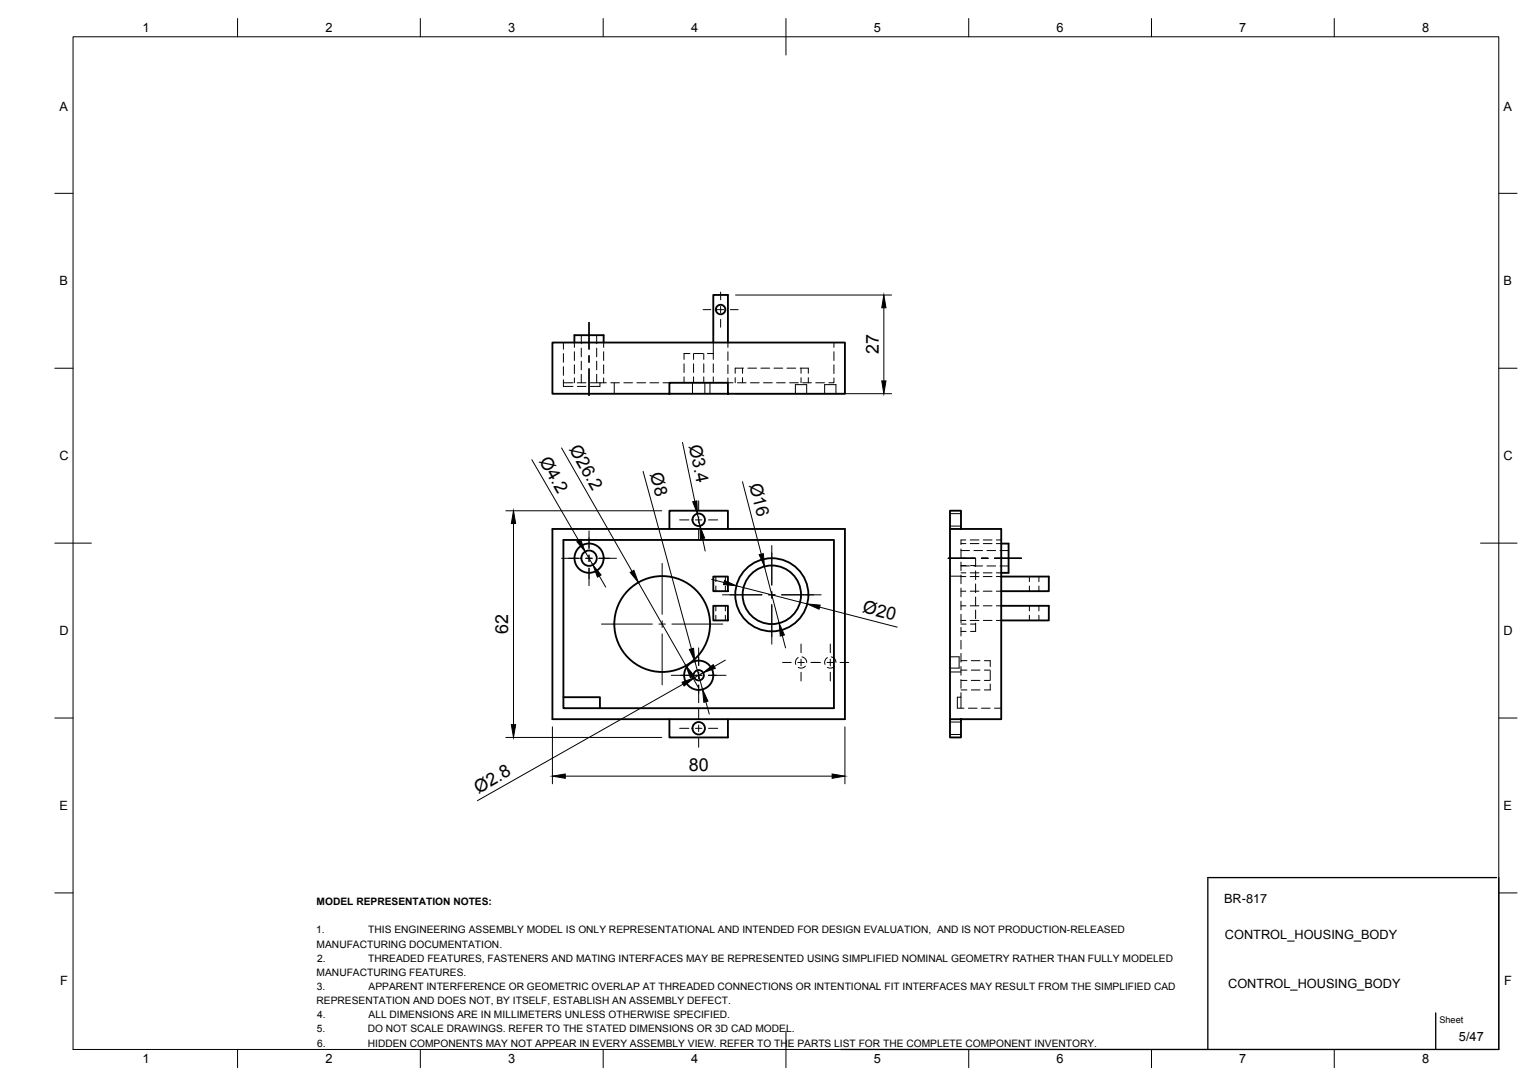
ISO-10303-21;
HEADER;
FILE_DESCRIPTION((''),'2;1');
FILE_NAME('CONTROL_HOUSING_BODY.step','2026-10-01T22:07:29-07:00',(''),(''),'','','');
FILE_SCHEMA (('AUTOMOTIVE_DESIGN { 1 0 10303 214 3 1 1 }'));
ENDSEC;
DATA;
#10=MECHANICAL_DESIGN_GEOMETRIC_PRESENTATION_REPRESENTATION('',(#543),#15484);
#473=SHAPE_REPRESENTATION_RELATIONSHIP('SRR','None',#15620,#508) ;
#508=ADVANCED_BREP_SHAPE_REPRESENTATION('',(#585),#15444) ;
#543=STYLED_ITEM('',(#15833),#585) ;
#585=MANIFOLD_SOLID_BREP('CONTROL_HOUSING_BODY',#8252) ;
#626=CYLINDRICAL_SURFACE('',#8695,0.155) ;
#627=CYLINDRICAL_SURFACE('',#8699,0.155) ;
#628=CYLINDRICAL_SURFACE('',#8703,0.17) ;
#629=CYLINDRICAL_SURFACE('',#8711,0.17) ;
#630=CYLINDRICAL_SURFACE('',#8719,0.14) ;
#631=CYLINDRICAL_SURFACE('',#8722,0.4) ;
#632=CYLINDRICAL_SURFACE('',#8726,0.8) ;
#633=CYLINDRICAL_SURFACE('',#8729,1.) ;
#634=CYLINDRICAL_SURFACE('',#8732,0.21) ;
#635=CYLINDRICAL_SURFACE('',#8735,0.4) ;
#636=CYLINDRICAL_SURFACE('',#8739,0.13) ;
#637=CYLINDRICAL_SURFACE('',#8742,0.13) ;
#638=CYLINDRICAL_SURFACE('',#8755,1.31) ;
#810=FACE_BOUND('',#1871,.T.) ;
#811=FACE_BOUND('',#1872,.T.) ;
#812=FACE_BOUND('',#1873,.T.) ;
#813=FACE_BOUND('',#1874,.T.) ;
#814=FACE_BOUND('',#1875,.T.) ;
#815=FACE_BOUND('',#1876,.T.) ;
#816=FACE_BOUND('',#1883,.T.) ;
#817=FACE_BOUND('',#1890,.T.) ;
#818=FACE_BOUND('',#1898,.T.) ;
#819=FACE_BOUND('',#1903,.T.) ;
#820=FACE_BOUND('',#1907,.T.) ;
#821=FACE_BOUND('',#1913,.T.) ;
#822=FACE_BOUND('',#1916,.T.) ;
#823=FACE_BOUND('',#1920,.T.) ;
#824=FACE_BOUND('',#1923,.T.) ;
#825=FACE_BOUND('',#1930,.T.) ;
#826=FACE_BOUND('',#1932,.T.) ;
#827=FACE_BOUND('',#1933,.T.) ;
#828=FACE_BOUND('',#1934,.T.) ;
#829=FACE_BOUND('',#1935,.T.) ;
#830=FACE_BOUND('',#1936,.T.) ;
#885=CIRCLE('',#8691,0.4) ;
#886=CIRCLE('',#8692,0.4) ;
#887=CIRCLE('',#8693,1.31) ;
#888=CIRCLE('',#8694,1.) ;
#889=CIRCLE('',#8696,0.155) ;
#890=CIRCLE('',#8697,0.155) ;
#891=CIRCLE('',#8700,0.155) ;
#892=CIRCLE('',#8701,0.155) ;
#893=CIRCLE('',#8704,0.17) ;
#894=CIRCLE('',#8705,0.17) ;
#895=CIRCLE('',#8712,0.17) ;
#896=CIRCLE('',#8713,0.17) ;
#897=CIRCLE('',#8720,0.14) ;
#898=CIRCLE('',#8721,0.14) ;
#899=CIRCLE('',#8723,0.4) ;
#900=CIRCLE('',#8727,0.8) ;
#901=CIRCLE('',#8728,0.8) ;
#902=CIRCLE('',#8730,1.) ;
#903=CIRCLE('',#8733,0.21) ;
#904=CIRCLE('',#8734,0.21) ;
#905=CIRCLE('',#8736,0.4) ;
#906=CIRCLE('',#8740,0.13) ;
#907=CIRCLE('',#8741,0.13) ;
#908=CIRCLE('',#8743,0.13) ;
#909=CIRCLE('',#8744,0.13) ;
#910=CIRCLE('',#8756,1.31) ;
#1365=FACE_OUTER_BOUND('',#1865,.T.) ;
#1366=FACE_OUTER_BOUND('',#1866,.T.) ;
#1367=FACE_OUTER_BOUND('',#1867,.T.) ;
#1368=FACE_OUTER_BOUND('',#1868,.T.) ;
#1369=FACE_OUTER_BOUND('',#1869,.T.) ;
#1370=FACE_OUTER_BOUND('',#1870,.T.) ;
#1371=FACE_OUTER_BOUND('',#1877,.T.) ;
#1372=FACE_OUTER_BOUND('',#1878,.T.) ;
#1373=FACE_OUTER_BOUND('',#1879,.T.) ;
#1374=FACE_OUTER_BOUND('',#1880,.T.) ;
#1375=FACE_OUTER_BOUND('',#1881,.T.) ;
#1376=FACE_OUTER_BOUND('',#1882,.T.) ;
#1377=FACE_OUTER_BOUND('',#1884,.T.) ;
#1378=FACE_OUTER_BOUND('',#1885,.T.) ;
#1379=FACE_OUTER_BOUND('',#1886,.T.) ;
#1380=FACE_OUTER_BOUND('',#1887,.T.) ;
#1381=FACE_OUTER_BOUND('',#1888,.T.) ;
#1382=FACE_OUTER_BOUND('',#1889,.T.) ;
#1383=FACE_OUTER_BOUND('',#1891,.T.) ;
#1384=FACE_OUTER_BOUND('',#1892,.T.) ;
#1385=FACE_OUTER_BOUND('',#1893,.T.) ;
#1386=FACE_OUTER_BOUND('',#1894,.T.) ;
#1387=FACE_OUTER_BOUND('',#1895,.T.) ;
#1388=FACE_OUTER_BOUND('',#1896,.T.) ;
#1389=FACE_OUTER_BOUND('',#1897,.T.) ;
#1390=FACE_OUTER_BOUND('',#1899,.T.) ;
#1391=FACE_OUTER_BOUND('',#1900,.T.) ;
#1392=FACE_OUTER_BOUND('',#1901,.T.) ;
#1393=FACE_OUTER_BOUND('',#1902,.T.) ;
#1394=FACE_OUTER_BOUND('',#1904,.T.) ;
#1395=FACE_OUTER_BOUND('',#1905,.T.) ;
#1396=FACE_OUTER_BOUND('',#1906,.T.) ;
#1397=FACE_OUTER_BOUND('',#1908,.T.) ;
#1398=FACE_OUTER_BOUND('',#1909,.T.) ;
#1399=FACE_OUTER_BOUND('',#1910,.T.) ;
#1400=FACE_OUTER_BOUND('',#1911,.T.) ;
#1401=FACE_OUTER_BOUND('',#1912,.T.) ;
#1402=FACE_OUTER_BOUND('',#1914,.T.) ;
#1403=FACE_OUTER_BOUND('',#1915,.T.) ;
#1404=FACE_OUTER_BOUND('',#1917,.T.) ;
#1405=FACE_OUTER_BOUND('',#1918,.T.) ;
#1406=FACE_OUTER_BOUND('',#1919,.T.) ;
#1407=FACE_OUTER_BOUND('',#1921,.T.) ;
#1408=FACE_OUTER_BOUND('',#1922,.T.) ;
#1409=FACE_OUTER_BOUND('',#1924,.T.) ;
#1410=FACE_OUTER_BOUND('',#1925,.T.) ;
#1411=FACE_OUTER_BOUND('',#1926,.T.) ;
#1412=FACE_OUTER_BOUND('',#1927,.T.) ;
#1413=FACE_OUTER_BOUND('',#1928,.T.) ;
#1414=FACE_OUTER_BOUND('',#1929,.T.) ;
#1415=FACE_OUTER_BOUND('',#1931,.T.) ;
#1416=FACE_OUTER_BOUND('',#1937,.T.) ;
#1417=FACE_OUTER_BOUND('',#1938,.T.) ;
#1865=EDGE_LOOP('',(#5273,#5274,#5275,#5276)) ;
#1866=EDGE_LOOP('',(#5277,#5278,#5279,#5280,#5281,#5282)) ;
#1867=EDGE_LOOP('',(#5283,#5284,#5285,#5286,#5287,#5288)) ;
#1868=EDGE_LOOP('',(#5289,#5290,#5291,#5292)) ;
#1869=EDGE_LOOP('',(#5293,#5294,#5295,#5296)) ;
#1870=EDGE_LOOP('',(#5297,#5298,#5299,#5300,#5301,#5302)) ;
#1871=EDGE_LOOP('',(#5303)) ;
#1872=EDGE_LOOP('',(#5304)) ;
#1873=EDGE_LOOP('',(#5305,#5306,#5307,#5308)) ;
#1874=EDGE_LOOP('',(#5309,#5310,#5311,#5312)) ;
#1875=EDGE_LOOP('',(#5313)) ;
#1876=EDGE_LOOP('',(#5314)) ;
#1877=EDGE_LOOP('',(#5315,#5316,#5317,#5318)) ;
#1878=EDGE_LOOP('',(#5319)) ;
#1879=EDGE_LOOP('',(#5320,#5321,#5322,#5323)) ;
#1880=EDGE_LOOP('',(#5324)) ;
#1881=EDGE_LOOP('',(#5325,#5326,#5327,#5328)) ;
#1882=EDGE_LOOP('',(#5329,#5330,#5331,#5332)) ;
#1883=EDGE_LOOP('',(#5333)) ;
#1884=EDGE_LOOP('',(#5334,#5335,#5336,#5337)) ;
#1885=EDGE_LOOP('',(#5338,#5339,#5340,#5341)) ;
#1886=EDGE_LOOP('',(#5342,#5343,#5344,#5345)) ;
#1887=EDGE_LOOP('',(#5346,#5347,#5348,#5349,#5350,#5351,#5352,#5353)) ;
#1888=EDGE_LOOP('',(#5354,#5355,#5356,#5357)) ;
#1889=EDGE_LOOP('',(#5358,#5359,#5360,#5361)) ;
#1890=EDGE_LOOP('',(#5362)) ;
#1891=EDGE_LOOP('',(#5363,#5364,#5365,#5366)) ;
#1892=EDGE_LOOP('',(#5367,#5368,#5369,#5370)) ;
#1893=EDGE_LOOP('',(#5371,#5372,#5373,#5374)) ;
#1894=EDGE_LOOP('',(#5375,#5376,#5377,#5378,#5379,#5380,#5381,#5382)) ;
#1895=EDGE_LOOP('',(#5383,#5384,#5385,#5386)) ;
#1896=EDGE_LOOP('',(#5387,#5388,#5389,#5390)) ;
#1897=EDGE_LOOP('',(#5391)) ;
#1898=EDGE_LOOP('',(#5392)) ;
#1899=EDGE_LOOP('',(#5393)) ;
#1900=EDGE_LOOP('',(#5394,#5395,#5396,#5397)) ;
#1901=EDGE_LOOP('',(#5398,#5399,#5400,#5401)) ;
#1902=EDGE_LOOP('',(#5402)) ;
#1903=EDGE_LOOP('',(#5403)) ;
#1904=EDGE_LOOP('',(#5404,#5405,#5406,#5407)) ;
#1905=EDGE_LOOP('',(#5408,#5409,#5410,#5411)) ;
#1906=EDGE_LOOP('',(#5412)) ;
#1907=EDGE_LOOP('',(#5413)) ;
#1908=EDGE_LOOP('',(#5414)) ;
#1909=EDGE_LOOP('',(#5415,#5416,#5417,#5418)) ;
#1910=EDGE_LOOP('',(#5419,#5420,#5421,#5422)) ;
#1911=EDGE_LOOP('',(#5423,#5424,#5425,#5426)) ;
#1912=EDGE_LOOP('',(#5427,#5428,#5429,#5430)) ;
#1913=EDGE_LOOP('',(#5431)) ;
#1914=EDGE_LOOP('',(#5432,#5433,#5434,#5435)) ;
#1915=EDGE_LOOP('',(#5436,#5437,#5438,#5439)) ;
#1916=EDGE_LOOP('',(#5440)) ;
#1917=EDGE_LOOP('',(#5441,#5442,#5443,#5444)) ;
#1918=EDGE_LOOP('',(#5445,#5446,#5447,#5448)) ;
#1919=EDGE_LOOP('',(#5449,#5450,#5451,#5452)) ;
#1920=EDGE_LOOP('',(#5453)) ;
#1921=EDGE_LOOP('',(#5454,#5455,#5456,#5457)) ;
#1922=EDGE_LOOP('',(#5458,#5459,#5460,#5461)) ;
#1923=EDGE_LOOP('',(#5462)) ;
#1924=EDGE_LOOP('',(#5463,#5464,#5465,#5466)) ;
#1925=EDGE_LOOP('',(#5467,#5468,#5469,#5470)) ;
#1926=EDGE_LOOP('',(#5471,#5472,#5473,#5474)) ;
#1927=EDGE_LOOP('',(#5475,#5476,#5477,#5478)) ;
#1928=EDGE_LOOP('',(#5479)) ;
#1929=EDGE_LOOP('',(#5480,#5481,#5482,#5483)) ;
#1930=EDGE_LOOP('',(#5484,#5485,#5486,#5487)) ;
#1931=EDGE_LOOP('',(#5488,#5489,#5490,#5491,#5492,#5493,#5494,#5495,#5496,
#5497,#5498,#5499)) ;
#1932=EDGE_LOOP('',(#5500)) ;
#1933=EDGE_LOOP('',(#5501)) ;
#1934=EDGE_LOOP('',(#5502)) ;
#1935=EDGE_LOOP('',(#5503)) ;
#1936=EDGE_LOOP('',(#5504)) ;
#1937=EDGE_LOOP('',(#5505,#5506,#5507,#5508)) ;
#1938=EDGE_LOOP('',(#5509,#5510,#5511,#5512)) ;
#2440=LINE('',#12891,#2914) ;
#2441=LINE('',#12893,#2915) ;
#2442=LINE('',#12895,#2916) ;
#2443=LINE('',#12896,#2917) ;
#2444=LINE('',#12899,#2918) ;
#2445=LINE('',#12901,#2919) ;
#2446=LINE('',#12903,#2920) ;
#2447=LINE('',#12905,#2921) ;
#2448=LINE('',#12906,#2922) ;
#2449=LINE('',#12909,#2923) ;
#2450=LINE('',#12911,#2924) ;
#2451=LINE('',#12913,#2925) ;
#2452=LINE('',#12914,#2926) ;
#2453=LINE('',#12917,#2927) ;
#2454=LINE('',#12918,#2928) ;
#2455=LINE('',#12920,#2929) ;
#2456=LINE('',#12923,#2930) ;
#2457=LINE('',#12924,#2931) ;
#2458=LINE('',#12931,#2932) ;
#2459=LINE('',#12933,#2933) ;
#2460=LINE('',#12935,#2934) ;
#2461=LINE('',#12936,#2935) ;
#2462=LINE('',#12939,#2936) ;
#2463=LINE('',#12941,#2937) ;
#2464=LINE('',#12943,#2938) ;
#2465=LINE('',#12944,#2939) ;
#2466=LINE('',#12953,#2940) ;
#2467=LINE('',#12960,#2941) ;
#2468=LINE('',#12967,#2942) ;
#2469=LINE('',#12972,#2943) ;
#2470=LINE('',#12974,#2944) ;
#2471=LINE('',#12976,#2945) ;
#2472=LINE('',#12977,#2946) ;
#2473=LINE('',#12980,#2947) ;
#2474=LINE('',#12982,#2948) ;
#2475=LINE('',#12983,#2949) ;
#2476=LINE('',#12986,#2950) ;
#2477=LINE('',#12987,#2951) ;
#2478=LINE('',#12990,#2952) ;
#2479=LINE('',#12991,#2953) ;
#2480=LINE('',#12994,#2954) ;
#2481=LINE('',#12996,#2955) ;
#2482=LINE('',#12998,#2956) ;
#2483=LINE('',#13000,#2957) ;
#2484=LINE('',#13001,#2958) ;
#2485=LINE('',#13006,#2959) ;
#2486=LINE('',#13011,#2960) ;
#2487=LINE('',#13013,#2961) ;
#2488=LINE('',#13015,#2962) ;
#2489=LINE('',#13016,#2963) ;
#2490=LINE('',#13019,#2964) ;
#2491=LINE('',#13021,#2965) ;
#2492=LINE('',#13022,#2966) ;
#2493=LINE('',#13025,#2967) ;
#2494=LINE('',#13026,#2968) ;
#2495=LINE('',#13029,#2969) ;
#2496=LINE('',#13030,#2970) ;
#2497=LINE('',#13033,#2971) ;
#2498=LINE('',#13035,#2972) ;
#2499=LINE('',#13037,#2973) ;
#2500=LINE('',#13039,#2974) ;
#2501=LINE('',#13040,#2975) ;
#2502=LINE('',#13045,#2976) ;
#2503=LINE('',#13050,#2977) ;
#2504=LINE('',#13057,#2978) ;
#2505=LINE('',#13062,#2979) ;
#2506=LINE('',#13068,#2980) ;
#2507=LINE('',#13073,#2981) ;
#2508=LINE('',#13080,#2982) ;
#2509=LINE('',#13086,#2983) ;
#2510=LINE('',#13091,#2984) ;
#2511=LINE('',#13093,#2985) ;
#2512=LINE('',#13095,#2986) ;
#2513=LINE('',#13096,#2987) ;
#2514=LINE('',#13098,#2988) ;
#2515=LINE('',#13099,#2989) ;
#2516=LINE('',#13101,#2990) ;
#2517=LINE('',#13103,#2991) ;
#2518=LINE('',#13108,#2992) ;
#2519=LINE('',#13110,#2993) ;
#2520=LINE('',#13112,#2994) ;
#2521=LINE('',#13113,#2995) ;
#2522=LINE('',#13115,#2996) ;
#2523=LINE('',#13116,#2997) ;
#2524=LINE('',#13118,#2998) ;
#2525=LINE('',#13120,#2999) ;
#2526=LINE('',#13125,#3000) ;
#2527=LINE('',#13128,#3001) ;
#2528=LINE('',#13129,#3002) ;
#2529=LINE('',#13131,#3003) ;
#2530=LINE('',#13134,#3004) ;
#2531=LINE('',#13135,#3005) ;
#2532=LINE('',#13137,#3006) ;
#2533=LINE('',#13138,#3007) ;
#2914=VECTOR('',#9933,1.) ;
#2915=VECTOR('',#9934,1.) ;
#2916=VECTOR('',#9935,1.) ;
#2917=VECTOR('',#9936,1.) ;
#2918=VECTOR('',#9939,1.) ;
#2919=VECTOR('',#9940,1.) ;
#2920=VECTOR('',#9941,1.) ;
#2921=VECTOR('',#9942,1.) ;
#2922=VECTOR('',#9943,1.) ;
#2923=VECTOR('',#9946,1.) ;
#2924=VECTOR('',#9947,1.) ;
#2925=VECTOR('',#9948,1.) ;
#2926=VECTOR('',#9949,1.) ;
#2927=VECTOR('',#9952,1.) ;
#2928=VECTOR('',#9953,1.) ;
#2929=VECTOR('',#9956,1.) ;
#2930=VECTOR('',#9959,1.) ;
#2931=VECTOR('',#9960,1.) ;
#2932=VECTOR('',#9965,1.) ;
#2933=VECTOR('',#9966,1.) ;
#2934=VECTOR('',#9967,1.) ;
#2935=VECTOR('',#9968,1.) ;
#2936=VECTOR('',#9969,1.) ;
#2937=VECTOR('',#9970,1.) ;
#2938=VECTOR('',#9971,1.) ;
#2939=VECTOR('',#9972,1.) ;
#2940=VECTOR('',#9981,0.155) ;
#2941=VECTOR('',#9990,0.155) ;
#2942=VECTOR('',#9999,0.17) ;
#2943=VECTOR('',#10004,1.) ;
#2944=VECTOR('',#10005,1.) ;
#2945=VECTOR('',#10006,1.) ;
#2946=VECTOR('',#10007,1.) ;
#2947=VECTOR('',#10010,1.) ;
#2948=VECTOR('',#10011,1.) ;
#2949=VECTOR('',#10012,1.) ;
#2950=VECTOR('',#10015,1.) ;
#2951=VECTOR('',#10016,1.) ;
#2952=VECTOR('',#10019,1.) ;
#2953=VECTOR('',#10020,1.) ;
#2954=VECTOR('',#10023,1.) ;
#2955=VECTOR('',#10024,1.) ;
#2956=VECTOR('',#10025,1.) ;
#2957=VECTOR('',#10026,1.) ;
#2958=VECTOR('',#10027,1.) ;
#2959=VECTOR('',#10032,0.17) ;
#2960=VECTOR('',#10037,1.) ;
#2961=VECTOR('',#10038,1.) ;
#2962=VECTOR('',#10039,1.) ;
#2963=VECTOR('',#10040,1.) ;
#2964=VECTOR('',#10043,1.) ;
#2965=VECTOR('',#10044,1.) ;
#2966=VECTOR('',#10045,1.) ;
#2967=VECTOR('',#10048,1.) ;
#2968=VECTOR('',#10049,1.) ;
#2969=VECTOR('',#10052,1.) ;
#2970=VECTOR('',#10053,1.) ;
#2971=VECTOR('',#10056,1.) ;
#2972=VECTOR('',#10057,1.) ;
#2973=VECTOR('',#10058,1.) ;
#2974=VECTOR('',#10059,1.) ;
#2975=VECTOR('',#10060,1.) ;
#2976=VECTOR('',#10065,0.14) ;
#2977=VECTOR('',#10072,0.4) ;
#2978=VECTOR('',#10081,0.8) ;
#2979=VECTOR('',#10088,1.) ;
#2980=VECTOR('',#10095,0.21) ;
#2981=VECTOR('',#10102,0.4) ;
#2982=VECTOR('',#10111,0.13) ;
#2983=VECTOR('',#10118,0.13) ;
#2984=VECTOR('',#10123,1.) ;
#2985=VECTOR('',#10124,1.) ;
#2986=VECTOR('',#10125,1.) ;
#2987=VECTOR('',#10126,1.) ;
#2988=VECTOR('',#10129,1.) ;
#2989=VECTOR('',#10130,1.) ;
#2990=VECTOR('',#10133,1.) ;
#2991=VECTOR('',#10136,1.) ;
#2992=VECTOR('',#10141,1.) ;
#2993=VECTOR('',#10142,1.) ;
#2994=VECTOR('',#10143,1.) ;
#2995=VECTOR('',#10144,1.) ;
#2996=VECTOR('',#10147,1.) ;
#2997=VECTOR('',#10148,1.) ;
#2998=VECTOR('',#10151,1.) ;
#2999=VECTOR('',#10154,1.) ;
#3000=VECTOR('',#10161,1.31) ;
#3001=VECTOR('',#10164,1.) ;
#3002=VECTOR('',#10165,1.) ;
#3003=VECTOR('',#10168,1.) ;
#3004=VECTOR('',#10173,1.) ;
#3005=VECTOR('',#10174,1.) ;
#3006=VECTOR('',#10177,1.) ;
#3007=VECTOR('',#10178,1.) ;
#3388=VERTEX_POINT('',#12889) ;
#3389=VERTEX_POINT('',#12890) ;
#3390=VERTEX_POINT('',#12892) ;
#3391=VERTEX_POINT('',#12894) ;
#3392=VERTEX_POINT('',#12898) ;
#3393=VERTEX_POINT('',#12900) ;
#3394=VERTEX_POINT('',#12902) ;
#3395=VERTEX_POINT('',#12904) ;
#3396=VERTEX_POINT('',#12908) ;
#3397=VERTEX_POINT('',#12910) ;
#3398=VERTEX_POINT('',#12912) ;
#3399=VERTEX_POINT('',#12916) ;
#3400=VERTEX_POINT('',#12922) ;
#3401=VERTEX_POINT('',#12925) ;
#3402=VERTEX_POINT('',#12927) ;
#3403=VERTEX_POINT('',#12929) ;
#3404=VERTEX_POINT('',#12930) ;
#3405=VERTEX_POINT('',#12932) ;
#3406=VERTEX_POINT('',#12934) ;
#3407=VERTEX_POINT('',#12937) ;
#3408=VERTEX_POINT('',#12938) ;
#3409=VERTEX_POINT('',#12940) ;
#3410=VERTEX_POINT('',#12942) ;
#3411=VERTEX_POINT('',#12945) ;
#3412=VERTEX_POINT('',#12947) ;
#3413=VERTEX_POINT('',#12950) ;
#3414=VERTEX_POINT('',#12952) ;
#3415=VERTEX_POINT('',#12957) ;
#3416=VERTEX_POINT('',#12959) ;
#3417=VERTEX_POINT('',#12964) ;
#3418=VERTEX_POINT('',#12966) ;
#3419=VERTEX_POINT('',#12970) ;
#3420=VERTEX_POINT('',#12971) ;
#3421=VERTEX_POINT('',#12973) ;
#3422=VERTEX_POINT('',#12975) ;
#3423=VERTEX_POINT('',#12979) ;
#3424=VERTEX_POINT('',#12981) ;
#3425=VERTEX_POINT('',#12985) ;
#3426=VERTEX_POINT('',#12989) ;
#3427=VERTEX_POINT('',#12993) ;
#3428=VERTEX_POINT('',#12995) ;
#3429=VERTEX_POINT('',#12997) ;
#3430=VERTEX_POINT('',#12999) ;
#3431=VERTEX_POINT('',#13003) ;
#3432=VERTEX_POINT('',#13005) ;
#3433=VERTEX_POINT('',#13009) ;
#3434=VERTEX_POINT('',#13010) ;
#3435=VERTEX_POINT('',#13012) ;
#3436=VERTEX_POINT('',#13014) ;
#3437=VERTEX_POINT('',#13018) ;
#3438=VERTEX_POINT('',#13020) ;
#3439=VERTEX_POINT('',#13024) ;
#3440=VERTEX_POINT('',#13028) ;
#3441=VERTEX_POINT('',#13032) ;
#3442=VERTEX_POINT('',#13034) ;
#3443=VERTEX_POINT('',#13036) ;
#3444=VERTEX_POINT('',#13038) ;
#3445=VERTEX_POINT('',#13042) ;
#3446=VERTEX_POINT('',#13044) ;
#3447=VERTEX_POINT('',#13048) ;
#3448=VERTEX_POINT('',#13054) ;
#3449=VERTEX_POINT('',#13056) ;
#3450=VERTEX_POINT('',#13060) ;
#3451=VERTEX_POINT('',#13065) ;
#3452=VERTEX_POINT('',#13067) ;
#3453=VERTEX_POINT('',#13071) ;
#3454=VERTEX_POINT('',#13077) ;
#3455=VERTEX_POINT('',#13079) ;
#3456=VERTEX_POINT('',#13083) ;
#3457=VERTEX_POINT('',#13085) ;
#3458=VERTEX_POINT('',#13089) ;
#3459=VERTEX_POINT('',#13090) ;
#3460=VERTEX_POINT('',#13092) ;
#3461=VERTEX_POINT('',#13094) ;
#3462=VERTEX_POINT('',#13106) ;
#3463=VERTEX_POINT('',#13107) ;
#3464=VERTEX_POINT('',#13109) ;
#3465=VERTEX_POINT('',#13111) ;
#3466=VERTEX_POINT('',#13123) ;
#3467=VERTEX_POINT('',#13127) ;
#4141=EDGE_CURVE('',#3388,#3389,#2440,.T.) ;
#4142=EDGE_CURVE('',#3390,#3388,#2441,.T.) ;
#4143=EDGE_CURVE('',#3391,#3390,#2442,.T.) ;
#4144=EDGE_CURVE('',#3389,#3391,#2443,.T.) ;
#4145=EDGE_CURVE('',#3392,#3391,#2444,.T.) ;
#4146=EDGE_CURVE('',#3393,#3392,#2445,.T.) ;
#4147=EDGE_CURVE('',#3393,#3394,#2446,.T.) ;
#4148=EDGE_CURVE('',#3394,#3395,#2447,.T.) ;
#4149=EDGE_CURVE('',#3395,#3389,#2448,.T.) ;
#4150=EDGE_CURVE('',#3396,#3390,#2449,.T.) ;
#4151=EDGE_CURVE('',#3396,#3397,#2450,.T.) ;
#4152=EDGE_CURVE('',#3398,#3397,#2451,.T.) ;
#4153=EDGE_CURVE('',#3392,#3398,#2452,.T.) ;
#4154=EDGE_CURVE('',#3399,#3388,#2453,.T.) ;
#4155=EDGE_CURVE('',#3396,#3399,#2454,.T.) ;
#4156=EDGE_CURVE('',#3399,#3395,#2455,.T.) ;
#4157=EDGE_CURVE('',#3400,#3394,#2456,.T.) ;
#4158=EDGE_CURVE('',#3397,#3400,#2457,.T.) ;
#4159=EDGE_CURVE('',#3401,#3401,#885,.T.) ;
#4160=EDGE_CURVE('',#3402,#3402,#886,.T.) ;
#4161=EDGE_CURVE('',#3403,#3404,#2458,.T.) ;
#4162=EDGE_CURVE('',#3404,#3405,#2459,.T.) ;
#4163=EDGE_CURVE('',#3405,#3406,#2460,.T.) ;
#4164=EDGE_CURVE('',#3406,#3403,#2461,.T.) ;
#4165=EDGE_CURVE('',#3407,#3408,#2462,.T.) ;
#4166=EDGE_CURVE('',#3408,#3409,#2463,.T.) ;
#4167=EDGE_CURVE('',#3409,#3410,#2464,.T.) ;
#4168=EDGE_CURVE('',#3410,#3407,#2465,.T.) ;
#4169=EDGE_CURVE('',#3411,#3411,#887,.T.) ;
#4170=EDGE_CURVE('',#3412,#3412,#888,.T.) ;
#4171=EDGE_CURVE('',#3413,#3413,#889,.T.) ;
#4172=EDGE_CURVE('',#3413,#3414,#2466,.T.) ;
#4173=EDGE_CURVE('',#3414,#3414,#890,.T.) ;
#4174=EDGE_CURVE('',#3415,#3415,#891,.T.) ;
#4175=EDGE_CURVE('',#3415,#3416,#2467,.T.) ;
#4176=EDGE_CURVE('',#3416,#3416,#892,.T.) ;
#4177=EDGE_CURVE('',#3417,#3417,#893,.T.) ;
#4178=EDGE_CURVE('',#3417,#3418,#2468,.T.) ;
#4179=EDGE_CURVE('',#3418,#3418,#894,.T.) ;
#4180=EDGE_CURVE('',#3419,#3420,#2469,.T.) ;
#4181=EDGE_CURVE('',#3421,#3420,#2470,.T.) ;
#4182=EDGE_CURVE('',#3421,#3422,#2471,.T.) ;
#4183=EDGE_CURVE('',#3422,#3419,#2472,.T.) ;
#4184=EDGE_CURVE('',#3422,#3423,#2473,.T.) ;
#4185=EDGE_CURVE('',#3424,#3423,#2474,.T.) ;
#4186=EDGE_CURVE('',#3419,#3424,#2475,.T.) ;
#4187=EDGE_CURVE('',#3425,#3421,#2476,.T.) ;
#4188=EDGE_CURVE('',#3423,#3425,#2477,.T.) ;
#4189=EDGE_CURVE('',#3426,#3424,#2478,.T.) ;
#4190=EDGE_CURVE('',#3420,#3426,#2479,.T.) ;
#4191=EDGE_CURVE('',#3427,#3426,#2480,.T.) ;
#4192=EDGE_CURVE('',#3428,#3427,#2481,.T.) ;
#4193=EDGE_CURVE('',#3429,#3428,#2482,.T.) ;
#4194=EDGE_CURVE('',#3429,#3430,#2483,.T.) ;
#4195=EDGE_CURVE('',#3425,#3430,#2484,.T.) ;
#4196=EDGE_CURVE('',#3431,#3431,#895,.T.) ;
#4197=EDGE_CURVE('',#3431,#3432,#2485,.T.) ;
#4198=EDGE_CURVE('',#3432,#3432,#896,.T.) ;
#4199=EDGE_CURVE('',#3433,#3434,#2486,.T.) ;
#4200=EDGE_CURVE('',#3434,#3435,#2487,.T.) ;
#4201=EDGE_CURVE('',#3435,#3436,#2488,.T.) ;
#4202=EDGE_CURVE('',#3433,#3436,#2489,.T.) ;
#4203=EDGE_CURVE('',#3435,#3437,#2490,.T.) ;
#4204=EDGE_CURVE('',#3438,#3437,#2491,.T.) ;
#4205=EDGE_CURVE('',#3436,#3438,#2492,.T.) ;
#4206=EDGE_CURVE('',#3434,#3439,#2493,.T.) ;
#4207=EDGE_CURVE('',#3437,#3439,#2494,.T.) ;
#4208=EDGE_CURVE('',#3440,#3433,#2495,.T.) ;
#4209=EDGE_CURVE('',#3439,#3440,#2496,.T.) ;
#4210=EDGE_CURVE('',#3441,#3438,#2497,.T.) ;
#4211=EDGE_CURVE('',#3442,#3441,#2498,.T.) ;
#4212=EDGE_CURVE('',#3443,#3442,#2499,.T.) ;
#4213=EDGE_CURVE('',#3443,#3444,#2500,.T.) ;
#4214=EDGE_CURVE('',#3440,#3444,#2501,.T.) ;
#4215=EDGE_CURVE('',#3445,#3445,#897,.T.) ;
#4216=EDGE_CURVE('',#3445,#3446,#2502,.T.) ;
#4217=EDGE_CURVE('',#3446,#3446,#898,.T.) ;
#4218=EDGE_CURVE('',#3447,#3447,#899,.T.) ;
#4219=EDGE_CURVE('',#3447,#3401,#2503,.T.) ;
#4220=EDGE_CURVE('',#3448,#3448,#900,.T.) ;
#4221=EDGE_CURVE('',#3448,#3449,#2504,.T.) ;
#4222=EDGE_CURVE('',#3449,#3449,#901,.T.) ;
#4223=EDGE_CURVE('',#3450,#3450,#902,.T.) ;
#4224=EDGE_CURVE('',#3450,#3412,#2505,.T.) ;
#4225=EDGE_CURVE('',#3451,#3451,#903,.T.) ;
#4226=EDGE_CURVE('',#3451,#3452,#2506,.T.) ;
#4227=EDGE_CURVE('',#3452,#3452,#904,.T.) ;
#4228=EDGE_CURVE('',#3453,#3453,#905,.T.) ;
#4229=EDGE_CURVE('',#3453,#3402,#2507,.T.) ;
#4230=EDGE_CURVE('',#3454,#3454,#906,.T.) ;
#4231=EDGE_CURVE('',#3454,#3455,#2508,.T.) ;
#4232=EDGE_CURVE('',#3455,#3455,#907,.T.) ;
#4233=EDGE_CURVE('',#3456,#3456,#908,.T.) ;
#4234=EDGE_CURVE('',#3456,#3457,#2509,.T.) ;
#4235=EDGE_CURVE('',#3457,#3457,#909,.T.) ;
#4236=EDGE_CURVE('',#3458,#3459,#2510,.T.) ;
#4237=EDGE_CURVE('',#3459,#3460,#2511,.T.) ;
#4238=EDGE_CURVE('',#3460,#3461,#2512,.T.) ;
#4239=EDGE_CURVE('',#3461,#3458,#2513,.T.) ;
#4240=EDGE_CURVE('',#3461,#3404,#2514,.T.) ;
#4241=EDGE_CURVE('',#3458,#3403,#2515,.T.) ;
#4242=EDGE_CURVE('',#3460,#3405,#2516,.T.) ;
#4243=EDGE_CURVE('',#3459,#3406,#2517,.T.) ;
#4244=EDGE_CURVE('',#3462,#3463,#2518,.T.) ;
#4245=EDGE_CURVE('',#3463,#3464,#2519,.T.) ;
#4246=EDGE_CURVE('',#3464,#3465,#2520,.T.) ;
#4247=EDGE_CURVE('',#3465,#3462,#2521,.T.) ;
#4248=EDGE_CURVE('',#3465,#3408,#2522,.T.) ;
#4249=EDGE_CURVE('',#3462,#3407,#2523,.T.) ;
#4250=EDGE_CURVE('',#3464,#3409,#2524,.T.) ;
#4251=EDGE_CURVE('',#3463,#3410,#2525,.T.) ;
#4252=EDGE_CURVE('',#3466,#3466,#910,.T.) ;
#4253=EDGE_CURVE('',#3466,#3411,#2526,.T.) ;
#4254=EDGE_CURVE('',#3398,#3467,#2527,.T.) ;
#4255=EDGE_CURVE('',#3467,#3400,#2528,.T.) ;
#4256=EDGE_CURVE('',#3467,#3393,#2529,.T.) ;
#4257=EDGE_CURVE('',#3428,#3443,#2530,.T.) ;
#4258=EDGE_CURVE('',#3442,#3429,#2531,.T.) ;
#4259=EDGE_CURVE('',#3444,#3427,#2532,.T.) ;
#4260=EDGE_CURVE('',#3430,#3441,#2533,.T.) ;
#5273=ORIENTED_EDGE('',*,*,#4141,.F.) ;
#5274=ORIENTED_EDGE('',*,*,#4142,.F.) ;
#5275=ORIENTED_EDGE('',*,*,#4143,.F.) ;
#5276=ORIENTED_EDGE('',*,*,#4144,.F.) ;
#5277=ORIENTED_EDGE('',*,*,#4144,.T.) ;
#5278=ORIENTED_EDGE('',*,*,#4145,.F.) ;
#5279=ORIENTED_EDGE('',*,*,#4146,.F.) ;
#5280=ORIENTED_EDGE('',*,*,#4147,.T.) ;
#5281=ORIENTED_EDGE('',*,*,#4148,.T.) ;
#5282=ORIENTED_EDGE('',*,*,#4149,.T.) ;
#5283=ORIENTED_EDGE('',*,*,#4143,.T.) ;
#5284=ORIENTED_EDGE('',*,*,#4150,.F.) ;
#5285=ORIENTED_EDGE('',*,*,#4151,.T.) ;
#5286=ORIENTED_EDGE('',*,*,#4152,.F.) ;
#5287=ORIENTED_EDGE('',*,*,#4153,.F.) ;
#5288=ORIENTED_EDGE('',*,*,#4145,.T.) ;
#5289=ORIENTED_EDGE('',*,*,#4142,.T.) ;
#5290=ORIENTED_EDGE('',*,*,#4154,.F.) ;
#5291=ORIENTED_EDGE('',*,*,#4155,.F.) ;
#5292=ORIENTED_EDGE('',*,*,#4150,.T.) ;
#5293=ORIENTED_EDGE('',*,*,#4141,.T.) ;
#5294=ORIENTED_EDGE('',*,*,#4149,.F.) ;
#5295=ORIENTED_EDGE('',*,*,#4156,.F.) ;
#5296=ORIENTED_EDGE('',*,*,#4154,.T.) ;
#5297=ORIENTED_EDGE('',*,*,#4155,.T.) ;
#5298=ORIENTED_EDGE('',*,*,#4156,.T.) ;
#5299=ORIENTED_EDGE('',*,*,#4148,.F.) ;
#5300=ORIENTED_EDGE('',*,*,#4157,.F.) ;
#5301=ORIENTED_EDGE('',*,*,#4158,.F.) ;
#5302=ORIENTED_EDGE('',*,*,#4151,.F.) ;
#5303=ORIENTED_EDGE('',*,*,#4159,.T.) ;
#5304=ORIENTED_EDGE('',*,*,#4160,.T.) ;
#5305=ORIENTED_EDGE('',*,*,#4161,.T.) ;
#5306=ORIENTED_EDGE('',*,*,#4162,.T.) ;
#5307=ORIENTED_EDGE('',*,*,#4163,.T.) ;
#5308=ORIENTED_EDGE('',*,*,#4164,.T.) ;
#5309=ORIENTED_EDGE('',*,*,#4165,.T.) ;
#5310=ORIENTED_EDGE('',*,*,#4166,.T.) ;
#5311=ORIENTED_EDGE('',*,*,#4167,.T.) ;
#5312=ORIENTED_EDGE('',*,*,#4168,.T.) ;
#5313=ORIENTED_EDGE('',*,*,#4169,.T.) ;
#5314=ORIENTED_EDGE('',*,*,#4170,.T.) ;
#5315=ORIENTED_EDGE('',*,*,#4171,.F.) ;
#5316=ORIENTED_EDGE('',*,*,#4172,.T.) ;
#5317=ORIENTED_EDGE('',*,*,#4173,.T.) ;
#5318=ORIENTED_EDGE('',*,*,#4172,.F.) ;
#5319=ORIENTED_EDGE('',*,*,#4173,.F.) ;
#5320=ORIENTED_EDGE('',*,*,#4174,.F.) ;
#5321=ORIENTED_EDGE('',*,*,#4175,.T.) ;
#5322=ORIENTED_EDGE('',*,*,#4176,.T.) ;
#5323=ORIENTED_EDGE('',*,*,#4175,.F.) ;
#5324=ORIENTED_EDGE('',*,*,#4176,.F.) ;
#5325=ORIENTED_EDGE('',*,*,#4177,.F.) ;
#5326=ORIENTED_EDGE('',*,*,#4178,.T.) ;
#5327=ORIENTED_EDGE('',*,*,#4179,.F.) ;
#5328=ORIENTED_EDGE('',*,*,#4178,.F.) ;
#5329=ORIENTED_EDGE('',*,*,#4180,.T.) ;
#5330=ORIENTED_EDGE('',*,*,#4181,.F.) ;
#5331=ORIENTED_EDGE('',*,*,#4182,.T.) ;
#5332=ORIENTED_EDGE('',*,*,#4183,.T.) ;
#5333=ORIENTED_EDGE('',*,*,#4179,.T.) ;
#5334=ORIENTED_EDGE('',*,*,#4184,.T.) ;
#5335=ORIENTED_EDGE('',*,*,#4185,.F.) ;
#5336=ORIENTED_EDGE('',*,*,#4186,.F.) ;
#5337=ORIENTED_EDGE('',*,*,#4183,.F.) ;
#5338=ORIENTED_EDGE('',*,*,#4187,.F.) ;
#5339=ORIENTED_EDGE('',*,*,#4188,.F.) ;
#5340=ORIENTED_EDGE('',*,*,#4184,.F.) ;
#5341=ORIENTED_EDGE('',*,*,#4182,.F.) ;
#5342=ORIENTED_EDGE('',*,*,#4186,.T.) ;
#5343=ORIENTED_EDGE('',*,*,#4189,.F.) ;
#5344=ORIENTED_EDGE('',*,*,#4190,.F.) ;
#5345=ORIENTED_EDGE('',*,*,#4180,.F.) ;
#5346=ORIENTED_EDGE('',*,*,#4187,.T.) ;
#5347=ORIENTED_EDGE('',*,*,#4181,.T.) ;
#5348=ORIENTED_EDGE('',*,*,#4190,.T.) ;
#5349=ORIENTED_EDGE('',*,*,#4191,.F.) ;
#5350=ORIENTED_EDGE('',*,*,#4192,.F.) ;
#5351=ORIENTED_EDGE('',*,*,#4193,.F.) ;
#5352=ORIENTED_EDGE('',*,*,#4194,.T.) ;
#5353=ORIENTED_EDGE('',*,*,#4195,.F.) ;
#5354=ORIENTED_EDGE('',*,*,#4196,.F.) ;
#5355=ORIENTED_EDGE('',*,*,#4197,.T.) ;
#5356=ORIENTED_EDGE('',*,*,#4198,.F.) ;
#5357=ORIENTED_EDGE('',*,*,#4197,.F.) ;
#5358=ORIENTED_EDGE('',*,*,#4199,.T.) ;
#5359=ORIENTED_EDGE('',*,*,#4200,.T.) ;
#5360=ORIENTED_EDGE('',*,*,#4201,.T.) ;
#5361=ORIENTED_EDGE('',*,*,#4202,.F.) ;
#5362=ORIENTED_EDGE('',*,*,#4198,.T.) ;
#5363=ORIENTED_EDGE('',*,*,#4203,.T.) ;
#5364=ORIENTED_EDGE('',*,*,#4204,.F.) ;
#5365=ORIENTED_EDGE('',*,*,#4205,.F.) ;
#5366=ORIENTED_EDGE('',*,*,#4201,.F.) ;
#5367=ORIENTED_EDGE('',*,*,#4206,.T.) ;
#5368=ORIENTED_EDGE('',*,*,#4207,.F.) ;
#5369=ORIENTED_EDGE('',*,*,#4203,.F.) ;
#5370=ORIENTED_EDGE('',*,*,#4200,.F.) ;
#5371=ORIENTED_EDGE('',*,*,#4208,.F.) ;
#5372=ORIENTED_EDGE('',*,*,#4209,.F.) ;
#5373=ORIENTED_EDGE('',*,*,#4206,.F.) ;
#5374=ORIENTED_EDGE('',*,*,#4199,.F.) ;
#5375=ORIENTED_EDGE('',*,*,#4208,.T.) ;
#5376=ORIENTED_EDGE('',*,*,#4202,.T.) ;
#5377=ORIENTED_EDGE('',*,*,#4205,.T.) ;
#5378=ORIENTED_EDGE('',*,*,#4210,.F.) ;
#5379=ORIENTED_EDGE('',*,*,#4211,.F.) ;
#5380=ORIENTED_EDGE('',*,*,#4212,.F.) ;
#5381=ORIENTED_EDGE('',*,*,#4213,.T.) ;
#5382=ORIENTED_EDGE('',*,*,#4214,.F.) ;
#5383=ORIENTED_EDGE('',*,*,#4215,.F.) ;
#5384=ORIENTED_EDGE('',*,*,#4216,.T.) ;
#5385=ORIENTED_EDGE('',*,*,#4217,.F.) ;
#5386=ORIENTED_EDGE('',*,*,#4216,.F.) ;
#5387=ORIENTED_EDGE('',*,*,#4218,.F.) ;
#5388=ORIENTED_EDGE('',*,*,#4219,.T.) ;
#5389=ORIENTED_EDGE('',*,*,#4159,.F.) ;
#5390=ORIENTED_EDGE('',*,*,#4219,.F.) ;
#5391=ORIENTED_EDGE('',*,*,#4218,.T.) ;
#5392=ORIENTED_EDGE('',*,*,#4217,.T.) ;
#5393=ORIENTED_EDGE('',*,*,#4215,.T.) ;
#5394=ORIENTED_EDGE('',*,*,#4220,.F.) ;
#5395=ORIENTED_EDGE('',*,*,#4221,.T.) ;
#5396=ORIENTED_EDGE('',*,*,#4222,.F.) ;
#5397=ORIENTED_EDGE('',*,*,#4221,.F.) ;
#5398=ORIENTED_EDGE('',*,*,#4223,.F.) ;
#5399=ORIENTED_EDGE('',*,*,#4224,.T.) ;
#5400=ORIENTED_EDGE('',*,*,#4170,.F.) ;
#5401=ORIENTED_EDGE('',*,*,#4224,.F.) ;
#5402=ORIENTED_EDGE('',*,*,#4223,.T.) ;
#5403=ORIENTED_EDGE('',*,*,#4222,.T.) ;
#5404=ORIENTED_EDGE('',*,*,#4225,.F.) ;
#5405=ORIENTED_EDGE('',*,*,#4226,.T.) ;
#5406=ORIENTED_EDGE('',*,*,#4227,.F.) ;
#5407=ORIENTED_EDGE('',*,*,#4226,.F.) ;
#5408=ORIENTED_EDGE('',*,*,#4228,.F.) ;
#5409=ORIENTED_EDGE('',*,*,#4229,.T.) ;
#5410=ORIENTED_EDGE('',*,*,#4160,.F.) ;
#5411=ORIENTED_EDGE('',*,*,#4229,.F.) ;
#5412=ORIENTED_EDGE('',*,*,#4228,.T.) ;
#5413=ORIENTED_EDGE('',*,*,#4227,.T.) ;
#5414=ORIENTED_EDGE('',*,*,#4220,.T.) ;
#5415=ORIENTED_EDGE('',*,*,#4230,.F.) ;
#5416=ORIENTED_EDGE('',*,*,#4231,.T.) ;
#5417=ORIENTED_EDGE('',*,*,#4232,.F.) ;
#5418=ORIENTED_EDGE('',*,*,#4231,.F.) ;
#5419=ORIENTED_EDGE('',*,*,#4233,.F.) ;
#5420=ORIENTED_EDGE('',*,*,#4234,.T.) ;
#5421=ORIENTED_EDGE('',*,*,#4235,.F.) ;
#5422=ORIENTED_EDGE('',*,*,#4234,.F.) ;
#5423=ORIENTED_EDGE('',*,*,#4236,.T.) ;
#5424=ORIENTED_EDGE('',*,*,#4237,.T.) ;
#5425=ORIENTED_EDGE('',*,*,#4238,.T.) ;
#5426=ORIENTED_EDGE('',*,*,#4239,.T.) ;
#5427=ORIENTED_EDGE('',*,*,#4240,.T.) ;
#5428=ORIENTED_EDGE('',*,*,#4161,.F.) ;
#5429=ORIENTED_EDGE('',*,*,#4241,.F.) ;
#5430=ORIENTED_EDGE('',*,*,#4239,.F.) ;
#5431=ORIENTED_EDGE('',*,*,#4233,.T.) ;
#5432=ORIENTED_EDGE('',*,*,#4242,.T.) ;
#5433=ORIENTED_EDGE('',*,*,#4162,.F.) ;
#5434=ORIENTED_EDGE('',*,*,#4240,.F.) ;
#5435=ORIENTED_EDGE('',*,*,#4238,.F.) ;
#5436=ORIENTED_EDGE('',*,*,#4243,.T.) ;
#5437=ORIENTED_EDGE('',*,*,#4163,.F.) ;
#5438=ORIENTED_EDGE('',*,*,#4242,.F.) ;
#5439=ORIENTED_EDGE('',*,*,#4237,.F.) ;
#5440=ORIENTED_EDGE('',*,*,#4235,.T.) ;
#5441=ORIENTED_EDGE('',*,*,#4241,.T.) ;
#5442=ORIENTED_EDGE('',*,*,#4164,.F.) ;
#5443=ORIENTED_EDGE('',*,*,#4243,.F.) ;
#5444=ORIENTED_EDGE('',*,*,#4236,.F.) ;
#5445=ORIENTED_EDGE('',*,*,#4244,.T.) ;
#5446=ORIENTED_EDGE('',*,*,#4245,.T.) ;
#5447=ORIENTED_EDGE('',*,*,#4246,.T.) ;
#5448=ORIENTED_EDGE('',*,*,#4247,.T.) ;
#5449=ORIENTED_EDGE('',*,*,#4248,.T.) ;
#5450=ORIENTED_EDGE('',*,*,#4165,.F.) ;
#5451=ORIENTED_EDGE('',*,*,#4249,.F.) ;
#5452=ORIENTED_EDGE('',*,*,#4247,.F.) ;
#5453=ORIENTED_EDGE('',*,*,#4230,.T.) ;
#5454=ORIENTED_EDGE('',*,*,#4250,.T.) ;
#5455=ORIENTED_EDGE('',*,*,#4166,.F.) ;
#5456=ORIENTED_EDGE('',*,*,#4248,.F.) ;
#5457=ORIENTED_EDGE('',*,*,#4246,.F.) ;
#5458=ORIENTED_EDGE('',*,*,#4251,.T.) ;
#5459=ORIENTED_EDGE('',*,*,#4167,.F.) ;
#5460=ORIENTED_EDGE('',*,*,#4250,.F.) ;
#5461=ORIENTED_EDGE('',*,*,#4245,.F.) ;
#5462=ORIENTED_EDGE('',*,*,#4232,.T.) ;
#5463=ORIENTED_EDGE('',*,*,#4249,.T.) ;
#5464=ORIENTED_EDGE('',*,*,#4168,.F.) ;
#5465=ORIENTED_EDGE('',*,*,#4251,.F.) ;
#5466=ORIENTED_EDGE('',*,*,#4244,.F.) ;
#5467=ORIENTED_EDGE('',*,*,#4252,.F.) ;
#5468=ORIENTED_EDGE('',*,*,#4253,.T.) ;
#5469=ORIENTED_EDGE('',*,*,#4169,.F.) ;
#5470=ORIENTED_EDGE('',*,*,#4253,.F.) ;
#5471=ORIENTED_EDGE('',*,*,#4254,.F.) ;
#5472=ORIENTED_EDGE('',*,*,#4152,.T.) ;
#5473=ORIENTED_EDGE('',*,*,#4158,.T.) ;
#5474=ORIENTED_EDGE('',*,*,#4255,.F.) ;
#5475=ORIENTED_EDGE('',*,*,#4256,.F.) ;
#5476=ORIENTED_EDGE('',*,*,#4255,.T.) ;
#5477=ORIENTED_EDGE('',*,*,#4157,.T.) ;
#5478=ORIENTED_EDGE('',*,*,#4147,.F.) ;
#5479=ORIENTED_EDGE('',*,*,#4225,.T.) ;
#5480=ORIENTED_EDGE('',*,*,#4257,.T.) ;
#5481=ORIENTED_EDGE('',*,*,#4212,.T.) ;
#5482=ORIENTED_EDGE('',*,*,#4258,.T.) ;
#5483=ORIENTED_EDGE('',*,*,#4193,.T.) ;
#5484=ORIENTED_EDGE('',*,*,#4146,.T.) ;
#5485=ORIENTED_EDGE('',*,*,#4153,.T.) ;
#5486=ORIENTED_EDGE('',*,*,#4254,.T.) ;
#5487=ORIENTED_EDGE('',*,*,#4256,.T.) ;
#5488=ORIENTED_EDGE('',*,*,#4259,.T.) ;
#5489=ORIENTED_EDGE('',*,*,#4191,.T.) ;
#5490=ORIENTED_EDGE('',*,*,#4189,.T.) ;
#5491=ORIENTED_EDGE('',*,*,#4185,.T.) ;
#5492=ORIENTED_EDGE('',*,*,#4188,.T.) ;
#5493=ORIENTED_EDGE('',*,*,#4195,.T.) ;
#5494=ORIENTED_EDGE('',*,*,#4260,.T.) ;
#5495=ORIENTED_EDGE('',*,*,#4210,.T.) ;
#5496=ORIENTED_EDGE('',*,*,#4204,.T.) ;
#5497=ORIENTED_EDGE('',*,*,#4207,.T.) ;
#5498=ORIENTED_EDGE('',*,*,#4209,.T.) ;
#5499=ORIENTED_EDGE('',*,*,#4214,.T.) ;
#5500=ORIENTED_EDGE('',*,*,#4171,.T.) ;
#5501=ORIENTED_EDGE('',*,*,#4174,.T.) ;
#5502=ORIENTED_EDGE('',*,*,#4177,.T.) ;
#5503=ORIENTED_EDGE('',*,*,#4196,.T.) ;
#5504=ORIENTED_EDGE('',*,*,#4252,.T.) ;
#5505=ORIENTED_EDGE('',*,*,#4211,.T.) ;
#5506=ORIENTED_EDGE('',*,*,#4260,.F.) ;
#5507=ORIENTED_EDGE('',*,*,#4194,.F.) ;
#5508=ORIENTED_EDGE('',*,*,#4258,.F.) ;
#5509=ORIENTED_EDGE('',*,*,#4192,.T.) ;
#5510=ORIENTED_EDGE('',*,*,#4259,.F.) ;
#5511=ORIENTED_EDGE('',*,*,#4213,.F.) ;
#5512=ORIENTED_EDGE('',*,*,#4257,.F.) ;
#7537=PLANE('',#8685) ;
#7538=PLANE('',#8686) ;
#7539=PLANE('',#8687) ;
#7540=PLANE('',#8688) ;
#7541=PLANE('',#8689) ;
#7542=PLANE('',#8690) ;
#7543=PLANE('',#8698) ;
#7544=PLANE('',#8702) ;
#7545=PLANE('',#8706) ;
#7546=PLANE('',#8707) ;
#7547=PLANE('',#8708) ;
#7548=PLANE('',#8709) ;
#7549=PLANE('',#8710) ;
#7550=PLANE('',#8714) ;
#7551=PLANE('',#8715) ;
#7552=PLANE('',#8716) ;
#7553=PLANE('',#8717) ;
#7554=PLANE('',#8718) ;
#7555=PLANE('',#8724) ;
#7556=PLANE('',#8725) ;
#7557=PLANE('',#8731) ;
#7558=PLANE('',#8737) ;
#7559=PLANE('',#8738) ;
#7560=PLANE('',#8745) ;
#7561=PLANE('',#8746) ;
#7562=PLANE('',#8747) ;
#7563=PLANE('',#8748) ;
#7564=PLANE('',#8749) ;
#7565=PLANE('',#8750) ;
#7566=PLANE('',#8751) ;
#7567=PLANE('',#8752) ;
#7568=PLANE('',#8753) ;
#7569=PLANE('',#8754) ;
#7570=PLANE('',#8757) ;
#7571=PLANE('',#8758) ;
#7572=PLANE('',#8759) ;
#7573=PLANE('',#8760) ;
#7574=PLANE('',#8761) ;
#7575=PLANE('',#8762) ;
#7576=PLANE('',#8763) ;
#7752=ADVANCED_FACE('',(#1365),#7537,.T.) ;
#7753=ADVANCED_FACE('',(#1366),#7538,.T.) ;
#7754=ADVANCED_FACE('',(#1367),#7539,.T.) ;
#7755=ADVANCED_FACE('',(#1368),#7540,.T.) ;
#7756=ADVANCED_FACE('',(#1369),#7541,.T.) ;
#7757=ADVANCED_FACE('',(#1370,#810,#811,#812,#813,#814,#815),#7542,.T.) ;
#7758=ADVANCED_FACE('',(#1371),#626,.F.) ;
#7759=ADVANCED_FACE('',(#1372),#7543,.F.) ;
#7760=ADVANCED_FACE('',(#1373),#627,.F.) ;
#7761=ADVANCED_FACE('',(#1374),#7544,.F.) ;
#7762=ADVANCED_FACE('',(#1375),#628,.F.) ;
#7763=ADVANCED_FACE('',(#1376,#816),#7545,.T.) ;
#7764=ADVANCED_FACE('',(#1377),#7546,.F.) ;
#7765=ADVANCED_FACE('',(#1378),#7547,.F.) ;
#7766=ADVANCED_FACE('',(#1379),#7548,.F.) ;
#7767=ADVANCED_FACE('',(#1380),#7549,.F.) ;
#7768=ADVANCED_FACE('',(#1381),#629,.F.) ;
#7769=ADVANCED_FACE('',(#1382,#817),#7550,.T.) ;
#7770=ADVANCED_FACE('',(#1383),#7551,.F.) ;
#7771=ADVANCED_FACE('',(#1384),#7552,.F.) ;
#7772=ADVANCED_FACE('',(#1385),#7553,.F.) ;
#7773=ADVANCED_FACE('',(#1386),#7554,.F.) ;
#7774=ADVANCED_FACE('',(#1387),#630,.F.) ;
#7775=ADVANCED_FACE('',(#1388),#631,.T.) ;
#7776=ADVANCED_FACE('',(#1389,#818),#7555,.T.) ;
#7777=ADVANCED_FACE('',(#1390),#7556,.T.) ;
#7778=ADVANCED_FACE('',(#1391),#632,.F.) ;
#7779=ADVANCED_FACE('',(#1392),#633,.T.) ;
#7780=ADVANCED_FACE('',(#1393,#819),#7557,.T.) ;
#7781=ADVANCED_FACE('',(#1394),#634,.F.) ;
#7782=ADVANCED_FACE('',(#1395),#635,.T.) ;
#7783=ADVANCED_FACE('',(#1396,#820),#7558,.T.) ;
#7784=ADVANCED_FACE('',(#1397),#7559,.T.) ;
#7785=ADVANCED_FACE('',(#1398),#636,.F.) ;
#7786=ADVANCED_FACE('',(#1399),#637,.F.) ;
#7787=ADVANCED_FACE('',(#1400),#7560,.T.) ;
#7788=ADVANCED_FACE('',(#1401,#821),#7561,.F.) ;
#7789=ADVANCED_FACE('',(#1402),#7562,.F.) ;
#7790=ADVANCED_FACE('',(#1403,#822),#7563,.F.) ;
#7791=ADVANCED_FACE('',(#1404),#7564,.F.) ;
#7792=ADVANCED_FACE('',(#1405),#7565,.T.) ;
#7793=ADVANCED_FACE('',(#1406,#823),#7566,.F.) ;
#7794=ADVANCED_FACE('',(#1407),#7567,.F.) ;
#7795=ADVANCED_FACE('',(#1408,#824),#7568,.F.) ;
#7796=ADVANCED_FACE('',(#1409),#7569,.F.) ;
#7797=ADVANCED_FACE('',(#1410),#638,.F.) ;
#7798=ADVANCED_FACE('',(#1411),#7570,.T.) ;
#7799=ADVANCED_FACE('',(#1412),#7571,.T.) ;
#7800=ADVANCED_FACE('',(#1413),#7572,.T.) ;
#7801=ADVANCED_FACE('',(#1414,#825),#7573,.T.) ;
#7802=ADVANCED_FACE('',(#1415,#826,#827,#828,#829,#830),#7574,.F.) ;
#7803=ADVANCED_FACE('',(#1416),#7575,.F.) ;
#7804=ADVANCED_FACE('',(#1417),#7576,.F.) ;
#8252=CLOSED_SHELL('',(#7752,#7753,#7754,#7755,#7756,#7757,#7758,#7759,
#7760,#7761,#7762,#7763,#7764,#7765,#7766,#7767,#7768,#7769,#7770,#7771,
#7772,#7773,#7774,#7775,#7776,#7777,#7778,#7779,#7780,#7781,#7782,#7783,
#7784,#7785,#7786,#7787,#7788,#7789,#7790,#7791,#7792,#7793,#7794,#7795,
#7796,#7797,#7798,#7799,#7800,#7801,#7802,#7803,#7804)) ;
#8684=AXIS2_PLACEMENT_3D('',#12887,#9929,#9930) ;
#8685=AXIS2_PLACEMENT_3D('',#12888,#9931,#9932) ;
#8686=AXIS2_PLACEMENT_3D('',#12897,#9937,#9938) ;
#8687=AXIS2_PLACEMENT_3D('',#12907,#9944,#9945) ;
#8688=AXIS2_PLACEMENT_3D('',#12915,#9950,#9951) ;
#8689=AXIS2_PLACEMENT_3D('',#12919,#9954,#9955) ;
#8690=AXIS2_PLACEMENT_3D('',#12921,#9957,#9958) ;
#8691=AXIS2_PLACEMENT_3D('',#12926,#9961,#9962) ;
#8692=AXIS2_PLACEMENT_3D('',#12928,#9963,#9964) ;
#8693=AXIS2_PLACEMENT_3D('',#12946,#9973,#9974) ;
#8694=AXIS2_PLACEMENT_3D('',#12948,#9975,#9976) ;
#8695=AXIS2_PLACEMENT_3D('',#12949,#9977,#9978) ;
#8696=AXIS2_PLACEMENT_3D('',#12951,#9979,#9980) ;
#8697=AXIS2_PLACEMENT_3D('',#12954,#9982,#9983) ;
#8698=AXIS2_PLACEMENT_3D('',#12955,#9984,#9985) ;
#8699=AXIS2_PLACEMENT_3D('',#12956,#9986,#9987) ;
#8700=AXIS2_PLACEMENT_3D('',#12958,#9988,#9989) ;
#8701=AXIS2_PLACEMENT_3D('',#12961,#9991,#9992) ;
#8702=AXIS2_PLACEMENT_3D('',#12962,#9993,#9994) ;
#8703=AXIS2_PLACEMENT_3D('',#12963,#9995,#9996) ;
#8704=AXIS2_PLACEMENT_3D('',#12965,#9997,#9998) ;
#8705=AXIS2_PLACEMENT_3D('',#12968,#10000,#10001) ;
#8706=AXIS2_PLACEMENT_3D('',#12969,#10002,#10003) ;
#8707=AXIS2_PLACEMENT_3D('',#12978,#10008,#10009) ;
#8708=AXIS2_PLACEMENT_3D('',#12984,#10013,#10014) ;
#8709=AXIS2_PLACEMENT_3D('',#12988,#10017,#10018) ;
#8710=AXIS2_PLACEMENT_3D('',#12992,#10021,#10022) ;
#8711=AXIS2_PLACEMENT_3D('',#13002,#10028,#10029) ;
#8712=AXIS2_PLACEMENT_3D('',#13004,#10030,#10031) ;
#8713=AXIS2_PLACEMENT_3D('',#13007,#10033,#10034) ;
#8714=AXIS2_PLACEMENT_3D('',#13008,#10035,#10036) ;
#8715=AXIS2_PLACEMENT_3D('',#13017,#10041,#10042) ;
#8716=AXIS2_PLACEMENT_3D('',#13023,#10046,#10047) ;
#8717=AXIS2_PLACEMENT_3D('',#13027,#10050,#10051) ;
#8718=AXIS2_PLACEMENT_3D('',#13031,#10054,#10055) ;
#8719=AXIS2_PLACEMENT_3D('',#13041,#10061,#10062) ;
#8720=AXIS2_PLACEMENT_3D('',#13043,#10063,#10064) ;
#8721=AXIS2_PLACEMENT_3D('',#13046,#10066,#10067) ;
#8722=AXIS2_PLACEMENT_3D('',#13047,#10068,#10069) ;
#8723=AXIS2_PLACEMENT_3D('',#13049,#10070,#10071) ;
#8724=AXIS2_PLACEMENT_3D('',#13051,#10073,#10074) ;
#8725=AXIS2_PLACEMENT_3D('',#13052,#10075,#10076) ;
#8726=AXIS2_PLACEMENT_3D('',#13053,#10077,#10078) ;
#8727=AXIS2_PLACEMENT_3D('',#13055,#10079,#10080) ;
#8728=AXIS2_PLACEMENT_3D('',#13058,#10082,#10083) ;
#8729=AXIS2_PLACEMENT_3D('',#13059,#10084,#10085) ;
#8730=AXIS2_PLACEMENT_3D('',#13061,#10086,#10087) ;
#8731=AXIS2_PLACEMENT_3D('',#13063,#10089,#10090) ;
#8732=AXIS2_PLACEMENT_3D('',#13064,#10091,#10092) ;
#8733=AXIS2_PLACEMENT_3D('',#13066,#10093,#10094) ;
#8734=AXIS2_PLACEMENT_3D('',#13069,#10096,#10097) ;
#8735=AXIS2_PLACEMENT_3D('',#13070,#10098,#10099) ;
#8736=AXIS2_PLACEMENT_3D('',#13072,#10100,#10101) ;
#8737=AXIS2_PLACEMENT_3D('',#13074,#10103,#10104) ;
#8738=AXIS2_PLACEMENT_3D('',#13075,#10105,#10106) ;
#8739=AXIS2_PLACEMENT_3D('',#13076,#10107,#10108) ;
#8740=AXIS2_PLACEMENT_3D('',#13078,#10109,#10110) ;
#8741=AXIS2_PLACEMENT_3D('',#13081,#10112,#10113) ;
#8742=AXIS2_PLACEMENT_3D('',#13082,#10114,#10115) ;
#8743=AXIS2_PLACEMENT_3D('',#13084,#10116,#10117) ;
#8744=AXIS2_PLACEMENT_3D('',#13087,#10119,#10120) ;
#8745=AXIS2_PLACEMENT_3D('',#13088,#10121,#10122) ;
#8746=AXIS2_PLACEMENT_3D('',#13097,#10127,#10128) ;
#8747=AXIS2_PLACEMENT_3D('',#13100,#10131,#10132) ;
#8748=AXIS2_PLACEMENT_3D('',#13102,#10134,#10135) ;
#8749=AXIS2_PLACEMENT_3D('',#13104,#10137,#10138) ;
#8750=AXIS2_PLACEMENT_3D('',#13105,#10139,#10140) ;
#8751=AXIS2_PLACEMENT_3D('',#13114,#10145,#10146) ;
#8752=AXIS2_PLACEMENT_3D('',#13117,#10149,#10150) ;
#8753=AXIS2_PLACEMENT_3D('',#13119,#10152,#10153) ;
#8754=AXIS2_PLACEMENT_3D('',#13121,#10155,#10156) ;
#8755=AXIS2_PLACEMENT_3D('',#13122,#10157,#10158) ;
#8756=AXIS2_PLACEMENT_3D('',#13124,#10159,#10160) ;
#8757=AXIS2_PLACEMENT_3D('',#13126,#10162,#10163) ;
#8758=AXIS2_PLACEMENT_3D('',#13130,#10166,#10167) ;
#8759=AXIS2_PLACEMENT_3D('',#13132,#10169,#10170) ;
#8760=AXIS2_PLACEMENT_3D('',#13133,#10171,#10172) ;
#8761=AXIS2_PLACEMENT_3D('',#13136,#10175,#10176) ;
#8762=AXIS2_PLACEMENT_3D('',#13139,#10179,#10180) ;
#8763=AXIS2_PLACEMENT_3D('',#13140,#10181,#10182) ;
#9929=DIRECTION('axis',(0.,0.,1.)) ;
#9930=DIRECTION('refdir',(1.,0.,0.)) ;
#9931=DIRECTION('center_axis',(0.,0.,1.)) ;
#9932=DIRECTION('ref_axis',(1.,0.,0.)) ;
#9933=DIRECTION('',(0.,-1.,0.)) ;
#9934=DIRECTION('',(1.,0.,0.)) ;
#9935=DIRECTION('',(0.,1.,0.)) ;
#9936=DIRECTION('',(-1.,0.,0.)) ;
#9937=DIRECTION('center_axis',(0.,1.,0.)) ;
#9938=DIRECTION('ref_axis',(0.,0.,1.)) ;
#9939=DIRECTION('',(0.,0.,-1.)) ;
#9940=DIRECTION('',(-1.,0.,0.)) ;
#9941=DIRECTION('',(0.,0.,-1.)) ;
#9942=DIRECTION('',(-1.,0.,0.)) ;
#9943=DIRECTION('',(0.,0.,-1.)) ;
#9944=DIRECTION('center_axis',(1.,0.,0.)) ;
#9945=DIRECTION('ref_axis',(0.,0.,-1.)) ;
#9946=DIRECTION('',(0.,0.,-1.)) ;
#9947=DIRECTION('',(0.,1.,0.)) ;
#9948=DIRECTION('',(0.,0.,-1.)) ;
#9949=DIRECTION('',(0.,1.,0.)) ;
#9950=DIRECTION('center_axis',(0.,-1.,0.)) ;
#9951=DIRECTION('ref_axis',(0.,0.,-1.)) ;
#9952=DIRECTION('',(0.,0.,-1.)) ;
#9953=DIRECTION('',(1.,0.,0.)) ;
#9954=DIRECTION('center_axis',(-1.,0.,0.)) ;
#9955=DIRECTION('ref_axis',(0.,0.,1.)) ;
#9956=DIRECTION('',(0.,-1.,0.)) ;
#9957=DIRECTION('center_axis',(0.,0.,1.)) ;
#9958=DIRECTION('ref_axis',(1.,0.,0.)) ;
#9959=DIRECTION('',(0.,-1.,0.)) ;
#9960=DIRECTION('',(1.,0.,0.)) ;
#9961=DIRECTION('center_axis',(0.,0.,-1.)) ;
#9962=DIRECTION('ref_axis',(1.,0.,0.)) ;
#9963=DIRECTION('center_axis',(0.,0.,-1.)) ;
#9964=DIRECTION('ref_axis',(1.,0.,0.)) ;
#9965=DIRECTION('',(-1.,0.,0.)) ;
#9966=DIRECTION('',(0.,1.,0.)) ;
#9967=DIRECTION('',(1.,0.,0.)) ;
#9968=DIRECTION('',(0.,-1.,0.)) ;
#9969=DIRECTION('',(-1.,0.,0.)) ;
#9970=DIRECTION('',(0.,1.,0.)) ;
#9971=DIRECTION('',(1.,0.,0.)) ;
#9972=DIRECTION('',(0.,-1.,0.)) ;
#9973=DIRECTION('center_axis',(0.,0.,-1.)) ;
#9974=DIRECTION('ref_axis',(1.,0.,0.)) ;
#9975=DIRECTION('center_axis',(0.,0.,-1.)) ;
#9976=DIRECTION('ref_axis',(1.,0.,0.)) ;
#9977=DIRECTION('center_axis',(0.,0.,1.)) ;
#9978=DIRECTION('ref_axis',(1.,0.,0.)) ;
#9979=DIRECTION('center_axis',(0.,0.,1.)) ;
#9980=DIRECTION('ref_axis',(1.,0.,0.)) ;
#9981=DIRECTION('',(0.,0.,1.)) ;
#9982=DIRECTION('center_axis',(0.,0.,1.)) ;
#9983=DIRECTION('ref_axis',(1.,0.,0.)) ;
#9984=DIRECTION('center_axis',(0.,0.,1.)) ;
#9985=DIRECTION('ref_axis',(1.,0.,0.)) ;
#9986=DIRECTION('center_axis',(0.,0.,1.)) ;
#9987=DIRECTION('ref_axis',(1.,0.,0.)) ;
#9988=DIRECTION('center_axis',(0.,0.,1.)) ;
#9989=DIRECTION('ref_axis',(1.,0.,0.)) ;
#9990=DIRECTION('',(0.,0.,1.)) ;
#9991=DIRECTION('center_axis',(0.,0.,1.)) ;
#9992=DIRECTION('ref_axis',(1.,0.,0.)) ;
#9993=DIRECTION('center_axis',(0.,0.,1.)) ;
#9994=DIRECTION('ref_axis',(1.,0.,0.)) ;
#9995=DIRECTION('center_axis',(0.,0.,1.)) ;
#9996=DIRECTION('ref_axis',(1.,0.,0.)) ;
#9997=DIRECTION('center_axis',(0.,0.,1.)) ;
#9998=DIRECTION('ref_axis',(1.,0.,0.)) ;
#9999=DIRECTION('',(0.,0.,1.)) ;
#10000=DIRECTION('center_axis',(0.,0.,-1.)) ;
#10001=DIRECTION('ref_axis',(1.,0.,0.)) ;
#10002=DIRECTION('center_axis',(0.,0.,1.)) ;
#10003=DIRECTION('ref_axis',(1.,0.,0.)) ;
#10004=DIRECTION('',(0.,1.,0.)) ;
#10005=DIRECTION('',(1.,0.,0.)) ;
#10006=DIRECTION('',(0.,-1.,0.)) ;
#10007=DIRECTION('',(1.,0.,0.)) ;
#10008=DIRECTION('center_axis',(0.,1.,0.)) ;
#10009=DIRECTION('ref_axis',(0.,0.,1.)) ;
#10010=DIRECTION('',(0.,0.,-1.)) ;
#10011=DIRECTION('',(-1.,0.,0.)) ;
#10012=DIRECTION('',(0.,0.,-1.)) ;
#10013=DIRECTION('center_axis',(1.,0.,0.)) ;
#10014=DIRECTION('ref_axis',(0.,0.,-1.)) ;
#10015=DIRECTION('',(0.,0.,1.)) ;
#10016=DIRECTION('',(0.,1.,0.)) ;
#10017=DIRECTION('center_axis',(-1.,0.,0.)) ;
#10018=DIRECTION('ref_axis',(0.,0.,1.)) ;
#10019=DIRECTION('',(0.,-1.,0.)) ;
#10020=DIRECTION('',(0.,0.,-1.)) ;
#10021=DIRECTION('center_axis',(0.,1.,0.)) ;
#10022=DIRECTION('ref_axis',(0.,0.,1.)) ;
#10023=DIRECTION('',(-1.,0.,0.)) ;
#10024=DIRECTION('',(0.,0.,-1.)) ;
#10025=DIRECTION('',(1.,0.,0.)) ;
#10026=DIRECTION('',(0.,0.,-1.)) ;
#10027=DIRECTION('',(-1.,0.,0.)) ;
#10028=DIRECTION('center_axis',(0.,0.,1.)) ;
#10029=DIRECTION('ref_axis',(1.,0.,0.)) ;
#10030=DIRECTION('center_axis',(0.,0.,1.)) ;
#10031=DIRECTION('ref_axis',(1.,0.,0.)) ;
#10032=DIRECTION('',(0.,0.,1.)) ;
#10033=DIRECTION('center_axis',(0.,0.,-1.)) ;
#10034=DIRECTION('ref_axis',(1.,0.,0.)) ;
#10035=DIRECTION('center_axis',(0.,0.,1.)) ;
#10036=DIRECTION('ref_axis',(1.,0.,0.)) ;
#10037=DIRECTION('',(0.,1.,0.)) ;
#10038=DIRECTION('',(-1.,0.,0.)) ;
#10039=DIRECTION('',(0.,-1.,0.)) ;
#10040=DIRECTION('',(-1.,0.,0.)) ;
#10041=DIRECTION('center_axis',(1.,0.,0.)) ;
#10042=DIRECTION('ref_axis',(0.,0.,-1.)) ;
#10043=DIRECTION('',(0.,0.,-1.)) ;
#10044=DIRECTION('',(0.,1.,0.)) ;
#10045=DIRECTION('',(0.,0.,-1.)) ;
#10046=DIRECTION('center_axis',(0.,-1.,0.)) ;
#10047=DIRECTION('ref_axis',(0.,0.,-1.)) ;
#10048=DIRECTION('',(0.,0.,-1.)) ;
#10049=DIRECTION('',(1.,0.,0.)) ;
#10050=DIRECTION('center_axis',(-1.,0.,0.)) ;
#10051=DIRECTION('ref_axis',(0.,0.,1.)) ;
#10052=DIRECTION('',(0.,0.,1.)) ;
#10053=DIRECTION('',(0.,-1.,0.)) ;
#10054=DIRECTION('center_axis',(0.,-1.,0.)) ;
#10055=DIRECTION('ref_axis',(0.,0.,-1.)) ;
#10056=DIRECTION('',(1.,0.,0.)) ;
#10057=DIRECTION('',(0.,0.,-1.)) ;
#10058=DIRECTION('',(-1.,0.,0.)) ;
#10059=DIRECTION('',(0.,0.,-1.)) ;
#10060=DIRECTION('',(1.,0.,0.)) ;
#10061=DIRECTION('center_axis',(0.,0.,1.)) ;
#10062=DIRECTION('ref_axis',(1.,0.,0.)) ;
#10063=DIRECTION('center_axis',(0.,0.,1.)) ;
#10064=DIRECTION('ref_axis',(1.,0.,0.)) ;
#10065=DIRECTION('',(0.,0.,1.)) ;
#10066=DIRECTION('center_axis',(0.,0.,-1.)) ;
#10067=DIRECTION('ref_axis',(1.,0.,0.)) ;
#10068=DIRECTION('center_axis',(0.,0.,1.)) ;
#10069=DIRECTION('ref_axis',(1.,0.,0.)) ;
#10070=DIRECTION('center_axis',(0.,0.,1.)) ;
#10071=DIRECTION('ref_axis',(1.,0.,0.)) ;
#10072=DIRECTION('',(0.,0.,-1.)) ;
#10073=DIRECTION('center_axis',(0.,0.,1.)) ;
#10074=DIRECTION('ref_axis',(1.,0.,0.)) ;
#10075=DIRECTION('center_axis',(0.,0.,1.)) ;
#10076=DIRECTION('ref_axis',(1.,0.,0.)) ;
#10077=DIRECTION('center_axis',(0.,0.,1.)) ;
#10078=DIRECTION('ref_axis',(1.,0.,0.)) ;
#10079=DIRECTION('center_axis',(0.,0.,1.)) ;
#10080=DIRECTION('ref_axis',(1.,0.,0.)) ;
#10081=DIRECTION('',(0.,0.,1.)) ;
#10082=DIRECTION('center_axis',(0.,0.,-1.)) ;
#10083=DIRECTION('ref_axis',(1.,0.,0.)) ;
#10084=DIRECTION('center_axis',(0.,0.,1.)) ;
#10085=DIRECTION('ref_axis',(1.,0.,0.)) ;
#10086=DIRECTION('center_axis',(0.,0.,1.)) ;
#10087=DIRECTION('ref_axis',(1.,0.,0.)) ;
#10088=DIRECTION('',(0.,0.,-1.)) ;
#10089=DIRECTION('center_axis',(0.,0.,1.)) ;
#10090=DIRECTION('ref_axis',(1.,0.,0.)) ;
#10091=DIRECTION('center_axis',(0.,0.,1.)) ;
#10092=DIRECTION('ref_axis',(1.,0.,0.)) ;
#10093=DIRECTION('center_axis',(0.,0.,1.)) ;
#10094=DIRECTION('ref_axis',(1.,0.,0.)) ;
#10095=DIRECTION('',(0.,0.,1.)) ;
#10096=DIRECTION('center_axis',(0.,0.,-1.)) ;
#10097=DIRECTION('ref_axis',(1.,0.,0.)) ;
#10098=DIRECTION('center_axis',(0.,0.,1.)) ;
#10099=DIRECTION('ref_axis',(1.,0.,0.)) ;
#10100=DIRECTION('center_axis',(0.,0.,1.)) ;
#10101=DIRECTION('ref_axis',(1.,0.,0.)) ;
#10102=DIRECTION('',(0.,0.,-1.)) ;
#10103=DIRECTION('center_axis',(0.,0.,1.)) ;
#10104=DIRECTION('ref_axis',(1.,0.,0.)) ;
#10105=DIRECTION('center_axis',(0.,0.,1.)) ;
#10106=DIRECTION('ref_axis',(1.,0.,0.)) ;
#10107=DIRECTION('center_axis',(0.,1.,0.)) ;
#10108=DIRECTION('ref_axis',(1.,0.,0.)) ;
#10109=DIRECTION('center_axis',(0.,1.,0.)) ;
#10110=DIRECTION('ref_axis',(1.,0.,0.)) ;
#10111=DIRECTION('',(0.,1.,0.)) ;
#10112=DIRECTION('center_axis',(0.,-1.,0.)) ;
#10113=DIRECTION('ref_axis',(1.,0.,0.)) ;
#10114=DIRECTION('center_axis',(0.,1.,0.)) ;
#10115=DIRECTION('ref_axis',(1.,0.,0.)) ;
#10116=DIRECTION('center_axis',(0.,1.,0.)) ;
#10117=DIRECTION('ref_axis',(1.,0.,0.)) ;
#10118=DIRECTION('',(0.,1.,0.)) ;
#10119=DIRECTION('center_axis',(0.,-1.,0.)) ;
#10120=DIRECTION('ref_axis',(1.,0.,0.)) ;
#10121=DIRECTION('center_axis',(0.,0.,1.)) ;
#10122=DIRECTION('ref_axis',(1.,0.,0.)) ;
#10123=DIRECTION('',(0.,1.,0.)) ;
#10124=DIRECTION('',(-1.,0.,0.)) ;
#10125=DIRECTION('',(0.,-1.,0.)) ;
#10126=DIRECTION('',(1.,0.,0.)) ;
#10127=DIRECTION('center_axis',(0.,1.,0.)) ;
#10128=DIRECTION('ref_axis',(0.,0.,1.)) ;
#10129=DIRECTION('',(0.,0.,-1.)) ;
#10130=DIRECTION('',(0.,0.,-1.)) ;
#10131=DIRECTION('center_axis',(1.,0.,0.)) ;
#10132=DIRECTION('ref_axis',(0.,0.,-1.)) ;
#10133=DIRECTION('',(0.,0.,-1.)) ;
#10134=DIRECTION('center_axis',(0.,-1.,0.)) ;
#10135=DIRECTION('ref_axis',(0.,0.,-1.)) ;
#10136=DIRECTION('',(0.,0.,-1.)) ;
#10137=DIRECTION('center_axis',(-1.,0.,0.)) ;
#10138=DIRECTION('ref_axis',(0.,0.,1.)) ;
#10139=DIRECTION('center_axis',(0.,0.,1.)) ;
#10140=DIRECTION('ref_axis',(1.,0.,0.)) ;
#10141=DIRECTION('',(0.,1.,0.)) ;
#10142=DIRECTION('',(-1.,0.,0.)) ;
#10143=DIRECTION('',(0.,-1.,0.)) ;
#10144=DIRECTION('',(1.,0.,0.)) ;
#10145=DIRECTION('center_axis',(0.,1.,0.)) ;
#10146=DIRECTION('ref_axis',(0.,0.,1.)) ;
#10147=DIRECTION('',(0.,0.,-1.)) ;
#10148=DIRECTION('',(0.,0.,-1.)) ;
#10149=DIRECTION('center_axis',(1.,0.,0.)) ;
#10150=DIRECTION('ref_axis',(0.,0.,-1.)) ;
#10151=DIRECTION('',(0.,0.,-1.)) ;
#10152=DIRECTION('center_axis',(0.,-1.,0.)) ;
#10153=DIRECTION('ref_axis',(0.,0.,-1.)) ;
#10154=DIRECTION('',(0.,0.,-1.)) ;
#10155=DIRECTION('center_axis',(-1.,0.,0.)) ;
#10156=DIRECTION('ref_axis',(0.,0.,1.)) ;
#10157=DIRECTION('center_axis',(0.,0.,1.)) ;
#10158=DIRECTION('ref_axis',(1.,0.,0.)) ;
#10159=DIRECTION('center_axis',(0.,0.,1.)) ;
#10160=DIRECTION('ref_axis',(1.,0.,0.)) ;
#10161=DIRECTION('',(0.,0.,1.)) ;
#10162=DIRECTION('center_axis',(0.,-1.,0.)) ;
#10163=DIRECTION('ref_axis',(0.,0.,-1.)) ;
#10164=DIRECTION('',(1.,0.,0.)) ;
#10165=DIRECTION('',(0.,0.,-1.)) ;
#10166=DIRECTION('center_axis',(-1.,0.,0.)) ;
#10167=DIRECTION('ref_axis',(0.,0.,1.)) ;
#10168=DIRECTION('',(0.,-1.,0.)) ;
#10169=DIRECTION('center_axis',(0.,0.,1.)) ;
#10170=DIRECTION('ref_axis',(1.,0.,0.)) ;
#10171=DIRECTION('center_axis',(0.,0.,1.)) ;
#10172=DIRECTION('ref_axis',(1.,0.,0.)) ;
#10173=DIRECTION('',(0.,1.,0.)) ;
#10174=DIRECTION('',(0.,-1.,0.)) ;
#10175=DIRECTION('center_axis',(0.,0.,1.)) ;
#10176=DIRECTION('ref_axis',(1.,0.,0.)) ;
#10177=DIRECTION('',(0.,-1.,0.)) ;
#10178=DIRECTION('',(0.,1.,0.)) ;
#10179=DIRECTION('center_axis',(1.,0.,0.)) ;
#10180=DIRECTION('ref_axis',(0.,0.,-1.)) ;
#10181=DIRECTION('center_axis',(-1.,0.,0.)) ;
#10182=DIRECTION('ref_axis',(0.,0.,1.)) ;
#12887=CARTESIAN_POINT('',(0.,0.,0.)) ;
#12888=CARTESIAN_POINT('Origin',(-3.2,-2.15,0.2)) ;
#12889=CARTESIAN_POINT('',(-2.7,-2.,0.2)) ;
#12890=CARTESIAN_POINT('',(-2.7,-2.3,0.2)) ;
#12891=CARTESIAN_POINT('',(-2.7,-2.15,0.2)) ;
#12892=CARTESIAN_POINT('',(-3.7,-2.,0.2)) ;
#12893=CARTESIAN_POINT('',(-3.2,-2.,0.2)) ;
#12894=CARTESIAN_POINT('',(-3.7,-2.3,0.2)) ;
#12895=CARTESIAN_POINT('',(-3.7,-1.075,0.2)) ;
#12896=CARTESIAN_POINT('',(-1.6,-2.3,0.2)) ;
#12897=CARTESIAN_POINT('Origin',(0.,-2.3,0.9)) ;
#12898=CARTESIAN_POINT('',(-3.7,-2.3,1.4)) ;
#12899=CARTESIAN_POINT('',(-3.7,-2.3,0.2)) ;
#12900=CARTESIAN_POINT('',(3.7,-2.3,1.4)) ;
#12901=CARTESIAN_POINT('',(0.,-2.3,1.4)) ;
#12902=CARTESIAN_POINT('',(3.7,-2.3,0.3)) ;
#12903=CARTESIAN_POINT('',(3.7,-2.3,0.9)) ;
#12904=CARTESIAN_POINT('',(-2.7,-2.3,0.3)) ;
#12905=CARTESIAN_POINT('',(0.,-2.3,0.3)) ;
#12906=CARTESIAN_POINT('',(-2.7,-2.3,0.2)) ;
#12907=CARTESIAN_POINT('Origin',(-3.7,0.,0.9)) ;
#12908=CARTESIAN_POINT('',(-3.7,-2.,0.3)) ;
#12909=CARTESIAN_POINT('',(-3.7,-2.,0.2)) ;
#12910=CARTESIAN_POINT('',(-3.7,2.3,0.3)) ;
#12911=CARTESIAN_POINT('',(-3.7,0.,0.3)) ;
#12912=CARTESIAN_POINT('',(-3.7,2.3,1.4)) ;
#12913=CARTESIAN_POINT('',(-3.7,2.3,0.9)) ;
#12914=CARTESIAN_POINT('',(-3.7,0.,1.4)) ;
#12915=CARTESIAN_POINT('Origin',(-3.2,-2.,0.2)) ;
#12916=CARTESIAN_POINT('',(-2.7,-2.,0.3)) ;
#12917=CARTESIAN_POINT('',(-2.7,-2.,0.2)) ;
#12918=CARTESIAN_POINT('',(-1.6,-2.,0.3)) ;
#12919=CARTESIAN_POINT('Origin',(-2.7,-2.15,0.2)) ;
#12920=CARTESIAN_POINT('',(-2.7,-1.075,0.3)) ;
#12921=CARTESIAN_POINT('Origin',(0.,0.,0.3)) ;
#12922=CARTESIAN_POINT('',(3.7,2.3,0.3)) ;
#12923=CARTESIAN_POINT('',(3.7,0.,0.3)) ;
#12924=CARTESIAN_POINT('',(0.,2.3,0.3)) ;
#12925=CARTESIAN_POINT('',(-0.4,-1.4,0.3)) ;
#12926=CARTESIAN_POINT('Origin',(0.,-1.4,0.3)) ;
#12927=CARTESIAN_POINT('',(-3.4,1.8,0.3)) ;
#12928=CARTESIAN_POINT('Origin',(-3.,1.8,0.3)) ;
#12929=CARTESIAN_POINT('',(0.8,0.9,0.3)) ;
#12930=CARTESIAN_POINT('',(0.4,0.9,0.3)) ;
#12931=CARTESIAN_POINT('',(0.3,0.9,0.3)) ;
#12932=CARTESIAN_POINT('',(0.4,1.3,0.3)) ;
#12933=CARTESIAN_POINT('',(0.4,0.55,0.3)) ;
#12934=CARTESIAN_POINT('',(0.8,1.3,0.3)) ;
#12935=CARTESIAN_POINT('',(0.3,1.3,0.3)) ;
#12936=CARTESIAN_POINT('',(0.8,0.55,0.3)) ;
#12937=CARTESIAN_POINT('',(0.8,0.1,0.3)) ;
#12938=CARTESIAN_POINT('',(0.4,0.1,0.3)) ;
#12939=CARTESIAN_POINT('',(0.3,0.1,0.3)) ;
#12940=CARTESIAN_POINT('',(0.4,0.5,0.3)) ;
#12941=CARTESIAN_POINT('',(0.4,0.15,0.3)) ;
#12942=CARTESIAN_POINT('',(0.8,0.5,0.3)) ;
#12943=CARTESIAN_POINT('',(0.3,0.5,0.3)) ;
#12944=CARTESIAN_POINT('',(0.8,0.15,0.3)) ;
#12945=CARTESIAN_POINT('',(-2.31,1.60428730688303E-16,0.3)) ;
#12946=CARTESIAN_POINT('Origin',(-1.,0.,0.3)) ;
#12947=CARTESIAN_POINT('',(1.,0.8,0.3)) ;
#12948=CARTESIAN_POINT('Origin',(2.,0.8,0.3)) ;
#12949=CARTESIAN_POINT('Origin',(3.6,-1.05,0.075)) ;
#12950=CARTESIAN_POINT('',(3.445,-1.05,0.)) ;
#12951=CARTESIAN_POINT('Origin',(3.6,-1.05,0.)) ;
#12952=CARTESIAN_POINT('',(3.445,-1.05,0.25)) ;
#12953=CARTESIAN_POINT('',(3.445,-1.05,0.075)) ;
#12954=CARTESIAN_POINT('Origin',(3.6,-1.05,0.25)) ;
#12955=CARTESIAN_POINT('Origin',(3.6,-1.05,0.25)) ;
#12956=CARTESIAN_POINT('Origin',(2.8,-1.05,0.075)) ;
#12957=CARTESIAN_POINT('',(2.645,-1.05,0.)) ;
#12958=CARTESIAN_POINT('Origin',(2.8,-1.05,0.)) ;
#12959=CARTESIAN_POINT('',(2.645,-1.05,0.25)) ;
#12960=CARTESIAN_POINT('',(2.645,-1.05,0.075)) ;
#12961=CARTESIAN_POINT('Origin',(2.8,-1.05,0.25)) ;
#12962=CARTESIAN_POINT('Origin',(2.8,-1.05,0.25)) ;
#12963=CARTESIAN_POINT('Origin',(0.,-2.85,0.15)) ;
#12964=CARTESIAN_POINT('',(-0.17,-2.85,0.)) ;
#12965=CARTESIAN_POINT('Origin',(0.,-2.85,0.)) ;
#12966=CARTESIAN_POINT('',(-0.17,-2.85,0.3)) ;
#12967=CARTESIAN_POINT('',(-0.17,-2.85,0.15)) ;
#12968=CARTESIAN_POINT('Origin',(0.,-2.85,0.3)) ;
#12969=CARTESIAN_POINT('Origin',(0.,-2.85,0.3)) ;
#12970=CARTESIAN_POINT('',(0.8,-3.1,0.3)) ;
#12971=CARTESIAN_POINT('',(0.8,-2.6,0.3)) ;
#12972=CARTESIAN_POINT('',(0.8,-2.85,0.3)) ;
#12973=CARTESIAN_POINT('',(-0.8,-2.6,0.3)) ;
#12974=CARTESIAN_POINT('',(0.,-2.6,0.3)) ;
#12975=CARTESIAN_POINT('',(-0.8,-3.1,0.3)) ;
#12976=CARTESIAN_POINT('',(-0.8,-2.85,0.3)) ;
#12977=CARTESIAN_POINT('',(0.,-3.1,0.3)) ;
#12978=CARTESIAN_POINT('Origin',(0.,-3.1,0.15)) ;
#12979=CARTESIAN_POINT('',(-0.8,-3.1,0.)) ;
#12980=CARTESIAN_POINT('',(-0.8,-3.1,0.15)) ;
#12981=CARTESIAN_POINT('',(0.8,-3.1,0.)) ;
#12982=CARTESIAN_POINT('',(0.,-3.1,0.)) ;
#12983=CARTESIAN_POINT('',(0.8,-3.1,0.15)) ;
#12984=CARTESIAN_POINT('Origin',(-0.8,-2.85,0.15)) ;
#12985=CARTESIAN_POINT('',(-0.8,-2.6,0.)) ;
#12986=CARTESIAN_POINT('',(-0.8,-2.6,0.425)) ;
#12987=CARTESIAN_POINT('',(-0.8,-2.85,0.)) ;
#12988=CARTESIAN_POINT('Origin',(0.8,-2.85,0.15)) ;
#12989=CARTESIAN_POINT('',(0.8,-2.6,0.)) ;
#12990=CARTESIAN_POINT('',(0.8,-2.85,0.)) ;
#12991=CARTESIAN_POINT('',(0.8,-2.6,0.425)) ;
#12992=CARTESIAN_POINT('Origin',(0.,-2.6,0.7)) ;
#12993=CARTESIAN_POINT('',(4.,-2.6,0.)) ;
#12994=CARTESIAN_POINT('',(0.,-2.6,0.)) ;
#12995=CARTESIAN_POINT('',(4.,-2.6,1.4)) ;
#12996=CARTESIAN_POINT('',(4.,-2.6,0.7)) ;
#12997=CARTESIAN_POINT('',(-4.,-2.6,1.4)) ;
#12998=CARTESIAN_POINT('',(0.,-2.6,1.4)) ;
#12999=CARTESIAN_POINT('',(-4.,-2.6,0.)) ;
#13000=CARTESIAN_POINT('',(-4.,-2.6,0.7)) ;
#13001=CARTESIAN_POINT('',(0.,-2.6,0.)) ;
#13002=CARTESIAN_POINT('Origin',(0.,2.85,0.15)) ;
#13003=CARTESIAN_POINT('',(-0.17,2.85,0.)) ;
#13004=CARTESIAN_POINT('Origin',(0.,2.85,0.)) ;
#13005=CARTESIAN_POINT('',(-0.17,2.85,0.3)) ;
#13006=CARTESIAN_POINT('',(-0.17,2.85,0.15)) ;
#13007=CARTESIAN_POINT('Origin',(0.,2.85,0.3)) ;
#13008=CARTESIAN_POINT('Origin',(0.,2.85,0.3)) ;
#13009=CARTESIAN_POINT('',(0.8,2.6,0.3)) ;
#13010=CARTESIAN_POINT('',(0.8,3.1,0.3)) ;
#13011=CARTESIAN_POINT('',(0.8,2.85,0.3)) ;
#13012=CARTESIAN_POINT('',(-0.8,3.1,0.3)) ;
#13013=CARTESIAN_POINT('',(0.,3.1,0.3)) ;
#13014=CARTESIAN_POINT('',(-0.8,2.6,0.3)) ;
#13015=CARTESIAN_POINT('',(-0.8,2.85,0.3)) ;
#13016=CARTESIAN_POINT('',(0.,2.6,0.3)) ;
#13017=CARTESIAN_POINT('Origin',(-0.8,2.85,0.15)) ;
#13018=CARTESIAN_POINT('',(-0.8,3.1,0.)) ;
#13019=CARTESIAN_POINT('',(-0.8,3.1,0.15)) ;
#13020=CARTESIAN_POINT('',(-0.8,2.6,0.)) ;
#13021=CARTESIAN_POINT('',(-0.8,2.85,0.)) ;
#13022=CARTESIAN_POINT('',(-0.8,2.6,0.425)) ;
#13023=CARTESIAN_POINT('Origin',(0.,3.1,0.15)) ;
#13024=CARTESIAN_POINT('',(0.8,3.1,0.)) ;
#13025=CARTESIAN_POINT('',(0.8,3.1,0.15)) ;
#13026=CARTESIAN_POINT('',(0.,3.1,0.)) ;
#13027=CARTESIAN_POINT('Origin',(0.8,2.85,0.15)) ;
#13028=CARTESIAN_POINT('',(0.8,2.6,0.)) ;
#13029=CARTESIAN_POINT('',(0.8,2.6,0.425)) ;
#13030=CARTESIAN_POINT('',(0.8,2.85,0.)) ;
#13031=CARTESIAN_POINT('Origin',(0.,2.6,0.7)) ;
#13032=CARTESIAN_POINT('',(-4.,2.6,0.)) ;
#13033=CARTESIAN_POINT('',(0.,2.6,0.)) ;
#13034=CARTESIAN_POINT('',(-4.,2.6,1.4)) ;
#13035=CARTESIAN_POINT('',(-4.,2.6,0.7)) ;
#13036=CARTESIAN_POINT('',(4.,2.6,1.4)) ;
#13037=CARTESIAN_POINT('',(0.,2.6,1.4)) ;
#13038=CARTESIAN_POINT('',(4.,2.6,0.)) ;
#13039=CARTESIAN_POINT('',(4.,2.6,0.7)) ;
#13040=CARTESIAN_POINT('',(0.,2.6,0.)) ;
#13041=CARTESIAN_POINT('Origin',(0.,-1.4,0.7)) ;
#13042=CARTESIAN_POINT('',(-0.14,-1.4,0.3)) ;
#13043=CARTESIAN_POINT('Origin',(0.,-1.4,0.3)) ;
#13044=CARTESIAN_POINT('',(-0.14,-1.4,1.1)) ;
#13045=CARTESIAN_POINT('',(-0.14,-1.4,0.7)) ;
#13046=CARTESIAN_POINT('Origin',(0.,-1.4,1.1)) ;
#13047=CARTESIAN_POINT('Origin',(0.,-1.4,0.7)) ;
#13048=CARTESIAN_POINT('',(-0.4,-1.4,1.1)) ;
#13049=CARTESIAN_POINT('Origin',(0.,-1.4,1.1)) ;
#13050=CARTESIAN_POINT('',(-0.4,-1.4,0.7)) ;
#13051=CARTESIAN_POINT('Origin',(0.,-1.4,1.1)) ;
#13052=CARTESIAN_POINT('Origin',(0.,0.,0.3)) ;
#13053=CARTESIAN_POINT('Origin',(2.,0.8,0.5)) ;
#13054=CARTESIAN_POINT('',(1.2,0.8,0.3)) ;
#13055=CARTESIAN_POINT('Origin',(2.,0.8,0.3)) ;
#13056=CARTESIAN_POINT('',(1.2,0.8,0.7)) ;
#13057=CARTESIAN_POINT('',(1.2,0.8,0.5)) ;
#13058=CARTESIAN_POINT('Origin',(2.,0.8,0.7)) ;
#13059=CARTESIAN_POINT('Origin',(2.,0.8,0.5)) ;
#13060=CARTESIAN_POINT('',(1.,0.8,0.7)) ;
#13061=CARTESIAN_POINT('Origin',(2.,0.8,0.7)) ;
#13062=CARTESIAN_POINT('',(1.,0.8,0.5)) ;
#13063=CARTESIAN_POINT('Origin',(2.,0.8,0.7)) ;
#13064=CARTESIAN_POINT('Origin',(-3.,1.8,0.95)) ;
#13065=CARTESIAN_POINT('',(-3.21,1.8,0.3)) ;
#13066=CARTESIAN_POINT('Origin',(-3.,1.8,0.3)) ;
#13067=CARTESIAN_POINT('',(-3.21,1.8,1.6)) ;
#13068=CARTESIAN_POINT('',(-3.21,1.8,0.95)) ;
#13069=CARTESIAN_POINT('Origin',(-3.,1.8,1.6)) ;
#13070=CARTESIAN_POINT('Origin',(-3.,1.8,0.95)) ;
#13071=CARTESIAN_POINT('',(-3.4,1.8,1.6)) ;
#13072=CARTESIAN_POINT('Origin',(-3.,1.8,1.6)) ;
#13073=CARTESIAN_POINT('',(-3.4,1.8,0.95)) ;
#13074=CARTESIAN_POINT('Origin',(-3.,1.8,1.6)) ;
#13075=CARTESIAN_POINT('Origin',(0.,0.,0.3)) ;
#13076=CARTESIAN_POINT('Origin',(0.6,0.7,2.3)) ;
#13077=CARTESIAN_POINT('',(0.47,0.1,2.3)) ;
#13078=CARTESIAN_POINT('Origin',(0.6,0.1,2.3)) ;
#13079=CARTESIAN_POINT('',(0.47,0.5,2.3)) ;
#13080=CARTESIAN_POINT('',(0.47,0.7,2.3)) ;
#13081=CARTESIAN_POINT('Origin',(0.6,0.5,2.3)) ;
#13082=CARTESIAN_POINT('Origin',(0.6,0.7,2.3)) ;
#13083=CARTESIAN_POINT('',(0.47,0.9,2.3)) ;
#13084=CARTESIAN_POINT('Origin',(0.6,0.9,2.3)) ;
#13085=CARTESIAN_POINT('',(0.47,1.3,2.3)) ;
#13086=CARTESIAN_POINT('',(0.47,0.7,2.3)) ;
#13087=CARTESIAN_POINT('Origin',(0.6,1.3,2.3)) ;
#13088=CARTESIAN_POINT('Origin',(0.6,1.1,2.7)) ;
#13089=CARTESIAN_POINT('',(0.8,0.9,2.7)) ;
#13090=CARTESIAN_POINT('',(0.8,1.3,2.7)) ;
#13091=CARTESIAN_POINT('',(0.8,1.1,2.7)) ;
#13092=CARTESIAN_POINT('',(0.4,1.3,2.7)) ;
#13093=CARTESIAN_POINT('',(0.6,1.3,2.7)) ;
#13094=CARTESIAN_POINT('',(0.4,0.9,2.7)) ;
#13095=CARTESIAN_POINT('',(0.4,1.1,2.7)) ;
#13096=CARTESIAN_POINT('',(0.6,0.9,2.7)) ;
#13097=CARTESIAN_POINT('Origin',(0.6,0.9,1.5)) ;
#13098=CARTESIAN_POINT('',(0.4,0.9,1.5)) ;
#13099=CARTESIAN_POINT('',(0.8,0.9,1.5)) ;
#13100=CARTESIAN_POINT('Origin',(0.4,1.1,1.5)) ;
#13101=CARTESIAN_POINT('',(0.4,1.3,1.5)) ;
#13102=CARTESIAN_POINT('Origin',(0.6,1.3,1.5)) ;
#13103=CARTESIAN_POINT('',(0.8,1.3,1.5)) ;
#13104=CARTESIAN_POINT('Origin',(0.8,1.1,1.5)) ;
#13105=CARTESIAN_POINT('Origin',(0.6,0.3,2.7)) ;
#13106=CARTESIAN_POINT('',(0.8,0.1,2.7)) ;
#13107=CARTESIAN_POINT('',(0.8,0.5,2.7)) ;
#13108=CARTESIAN_POINT('',(0.8,0.3,2.7)) ;
#13109=CARTESIAN_POINT('',(0.4,0.5,2.7)) ;
#13110=CARTESIAN_POINT('',(0.6,0.5,2.7)) ;
#13111=CARTESIAN_POINT('',(0.4,0.1,2.7)) ;
#13112=CARTESIAN_POINT('',(0.4,0.3,2.7)) ;
#13113=CARTESIAN_POINT('',(0.6,0.1,2.7)) ;
#13114=CARTESIAN_POINT('Origin',(0.6,0.1,1.5)) ;
#13115=CARTESIAN_POINT('',(0.4,0.1,1.5)) ;
#13116=CARTESIAN_POINT('',(0.8,0.1,1.5)) ;
#13117=CARTESIAN_POINT('Origin',(0.4,0.3,1.5)) ;
#13118=CARTESIAN_POINT('',(0.4,0.5,1.5)) ;
#13119=CARTESIAN_POINT('Origin',(0.6,0.5,1.5)) ;
#13120=CARTESIAN_POINT('',(0.8,0.5,1.5)) ;
#13121=CARTESIAN_POINT('Origin',(0.8,0.3,1.5)) ;
#13122=CARTESIAN_POINT('Origin',(-1.,0.,0.15)) ;
#13123=CARTESIAN_POINT('',(-2.31,-1.60428730688303E-16,0.)) ;
#13124=CARTESIAN_POINT('Origin',(-1.,0.,0.)) ;
#13125=CARTESIAN_POINT('',(-2.31,-1.60428730688303E-16,0.15)) ;
#13126=CARTESIAN_POINT('Origin',(0.,2.3,0.9)) ;
#13127=CARTESIAN_POINT('',(3.7,2.3,1.4)) ;
#13128=CARTESIAN_POINT('',(0.,2.3,1.4)) ;
#13129=CARTESIAN_POINT('',(3.7,2.3,0.9)) ;
#13130=CARTESIAN_POINT('Origin',(3.7,0.,0.9)) ;
#13131=CARTESIAN_POINT('',(3.7,0.,1.4)) ;
#13132=CARTESIAN_POINT('Origin',(0.,0.,0.3)) ;
#13133=CARTESIAN_POINT('Origin',(0.,0.,1.4)) ;
#13134=CARTESIAN_POINT('',(4.,0.,1.4)) ;
#13135=CARTESIAN_POINT('',(-4.,0.,1.4)) ;
#13136=CARTESIAN_POINT('Origin',(0.,0.,0.)) ;
#13137=CARTESIAN_POINT('',(4.,0.,0.)) ;
#13138=CARTESIAN_POINT('',(-4.,0.,0.)) ;
#13139=CARTESIAN_POINT('Origin',(-4.,0.,0.7)) ;
#13140=CARTESIAN_POINT('Origin',(4.,0.,0.7)) ;
#15401=UNCERTAINTY_MEASURE_WITH_UNIT(LENGTH_MEASURE(0.001),#15485,
'DISTANCE_ACCURACY_VALUE',
'Maximum model space distance between geometric entities at asserted c
onnectivities') ;
#15441=UNCERTAINTY_MEASURE_WITH_UNIT(LENGTH_MEASURE(0.001),#15485,
'DISTANCE_ACCURACY_VALUE',
'Maximum model space distance between geometric entities at asserted c
onnectivities') ;
#15444=(
GEOMETRIC_REPRESENTATION_CONTEXT(3)
GLOBAL_UNCERTAINTY_ASSIGNED_CONTEXT((#15401))
GLOBAL_UNIT_ASSIGNED_CONTEXT((#15485,#15487,#15488))
REPRESENTATION_CONTEXT('','3D')
) ;
#15484=(
GEOMETRIC_REPRESENTATION_CONTEXT(3)
GLOBAL_UNCERTAINTY_ASSIGNED_CONTEXT((#15441))
GLOBAL_UNIT_ASSIGNED_CONTEXT((#15485,#15487,#15488))
REPRESENTATION_CONTEXT('','3D')
) ;
#15485=(
LENGTH_UNIT()
NAMED_UNIT(*)
SI_UNIT(.CENTI.,.METRE.)
) ;
#15487=(
NAMED_UNIT(*)
PLANE_ANGLE_UNIT()
SI_UNIT($,.RADIAN.)
) ;
#15488=(
NAMED_UNIT(*)
SI_UNIT($,.STERADIAN.)
SOLID_ANGLE_UNIT()
) ;
#15491=SHAPE_DEFINITION_REPRESENTATION(#15533,#15620) ;
#15533=PRODUCT_DEFINITION_SHAPE('',$,#15663) ;
#15620=SHAPE_REPRESENTATION('',(#8684),#15444) ;
#15660=PRODUCT_DEFINITION_CONTEXT('part definition',#15788,'design') ;
#15663=PRODUCT_DEFINITION('CONTROL_HOUSING_BODY',
'CONTROL_HOUSING_BODY',#15705,#15660) ;
#15705=PRODUCT_DEFINITION_FORMATION('',$,#15792) ;
#15788=APPLICATION_CONTEXT(
'Core Data for Automotive Mechanical Design Process') ;
#15789=PRODUCT_CONTEXT('part definition',#15788,'mechanical') ;
#15792=PRODUCT('CONTROL_HOUSING_BODY','CONTROL_HOUSING_BODY',$,(#15789)) ;
#15833=PRESENTATION_STYLE_ASSIGNMENT((#15845)) ;
#15845=SURFACE_STYLE_USAGE(.BOTH.,#15857) ;
#15857=SURFACE_SIDE_STYLE('',(#15869)) ;
#15869=SURFACE_STYLE_FILL_AREA(#15881) ;
#15881=FILL_AREA_STYLE('Nylon 6-6 (White)',(#15893)) ;
#15893=FILL_AREA_STYLE_COLOUR('Nylon 6-6 (White)',#15905) ;
#15905=COLOUR_RGB('Nylon 6-6 (White)', 0.31764706, 0.68627451, 0.89019608) ;
ENDSEC;
END-ISO-10303-21;
